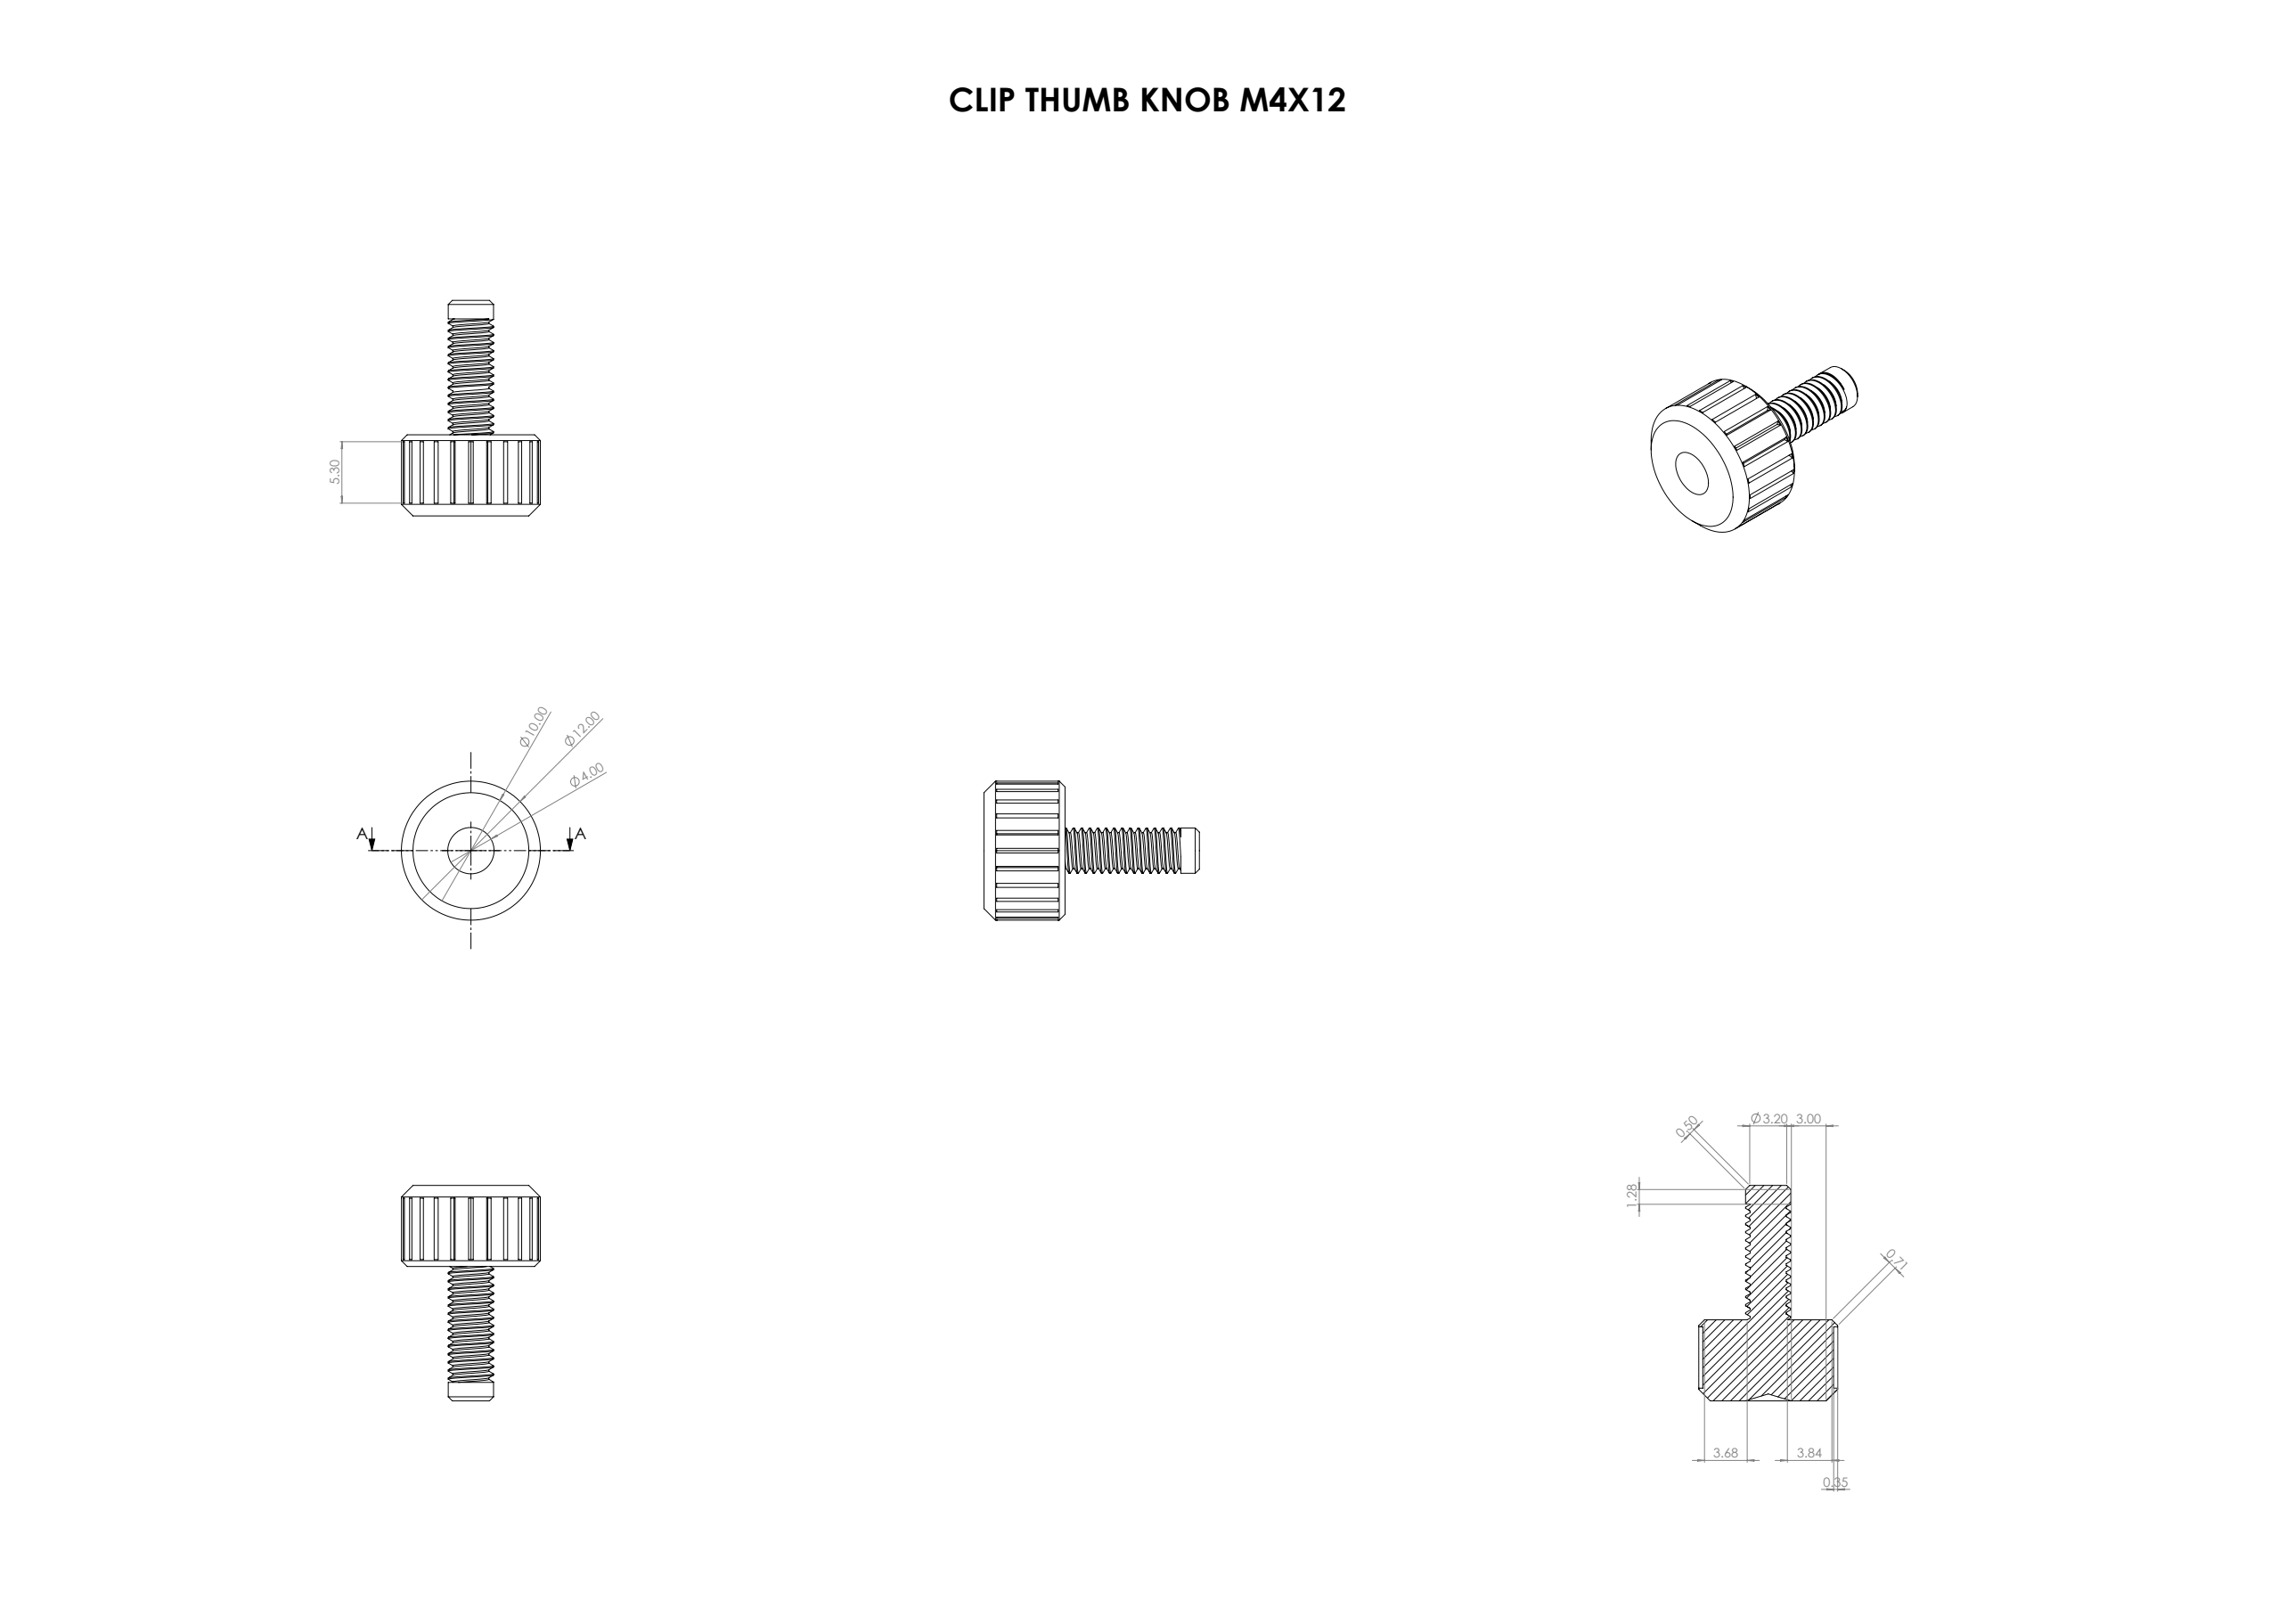
ISO-10303-21;
HEADER;
/* Generated by software containing ST-Developer
 * from STEP Tools, Inc. (www.steptools.com) 
 */

FILE_DESCRIPTION(
/* description */ (''),
/* implementation_level */ '2;1');

FILE_NAME(
/* name */ '11_Clip_Thumb_Knob_M4x12.step',
/* time_stamp */ '2026-10-19T22:59:19-07:00',
/* author */ (''),
/* organization */ (''),
/* preprocessor_version */ 'ST-DEVELOPER v20.2',
/* originating_system */ 'Autodesk Translation Framework v15.15.0.0',
/* authorisation */ '');

FILE_SCHEMA (('AUTOMOTIVE_DESIGN { 1 0 10303 214 3 1 1 }'));
ENDSEC;

DATA;
#10=MECHANICAL_DESIGN_GEOMETRIC_PRESENTATION_REPRESENTATION('',(#923),#53650);
#365=B_SPLINE_SURFACE_WITH_KNOTS('',3,3,((#37203,#37204,#37205,#37206,#37207,
#37208,#37209,#37210,#37211,#37212,#37213,#37214,#37215,#37216,#37217,#37218,
#37219,#37220,#37221,#37222,#37223,#37224,#37225,#37226,#37227,#37228,#37229,
#37230,#37231,#37232,#37233,#37234,#37235,#37236,#37237,#37238,#37239,#37240,
#37241,#37242,#37243,#37244,#37245,#37246,#37247,#37248,#37249,#37250,#37251,
#37252,#37253,#37254,#37255,#37256,#37257,#37258,#37259,#37260,#37261,#37262,
#37263,#37264,#37265,#37266,#37267,#37268,#37269,#37270,#37271,#37272,#37273,
#37274,#37275,#37276,#37277,#37278,#37279,#37280,#37281,#37282,#37283,#37284,
#37285,#37286,#37287,#37288,#37289,#37290,#37291,#37292,#37293,#37294,#37295,
#37296,#37297),(#37298,#37299,#37300,#37301,#37302,#37303,#37304,#37305,
#37306,#37307,#37308,#37309,#37310,#37311,#37312,#37313,#37314,#37315,#37316,
#37317,#37318,#37319,#37320,#37321,#37322,#37323,#37324,#37325,#37326,#37327,
#37328,#37329,#37330,#37331,#37332,#37333,#37334,#37335,#37336,#37337,#37338,
#37339,#37340,#37341,#37342,#37343,#37344,#37345,#37346,#37347,#37348,#37349,
#37350,#37351,#37352,#37353,#37354,#37355,#37356,#37357,#37358,#37359,#37360,
#37361,#37362,#37363,#37364,#37365,#37366,#37367,#37368,#37369,#37370,#37371,
#37372,#37373,#37374,#37375,#37376,#37377,#37378,#37379,#37380,#37381,#37382,
#37383,#37384,#37385,#37386,#37387,#37388,#37389,#37390,#37391,#37392),
(#37393,#37394,#37395,#37396,#37397,#37398,#37399,#37400,#37401,#37402,
#37403,#37404,#37405,#37406,#37407,#37408,#37409,#37410,#37411,#37412,#37413,
#37414,#37415,#37416,#37417,#37418,#37419,#37420,#37421,#37422,#37423,#37424,
#37425,#37426,#37427,#37428,#37429,#37430,#37431,#37432,#37433,#37434,#37435,
#37436,#37437,#37438,#37439,#37440,#37441,#37442,#37443,#37444,#37445,#37446,
#37447,#37448,#37449,#37450,#37451,#37452,#37453,#37454,#37455,#37456,#37457,
#37458,#37459,#37460,#37461,#37462,#37463,#37464,#37465,#37466,#37467,#37468,
#37469,#37470,#37471,#37472,#37473,#37474,#37475,#37476,#37477,#37478,#37479,
#37480,#37481,#37482,#37483,#37484,#37485,#37486,#37487),(#37488,#37489,
#37490,#37491,#37492,#37493,#37494,#37495,#37496,#37497,#37498,#37499,#37500,
#37501,#37502,#37503,#37504,#37505,#37506,#37507,#37508,#37509,#37510,#37511,
#37512,#37513,#37514,#37515,#37516,#37517,#37518,#37519,#37520,#37521,#37522,
#37523,#37524,#37525,#37526,#37527,#37528,#37529,#37530,#37531,#37532,#37533,
#37534,#37535,#37536,#37537,#37538,#37539,#37540,#37541,#37542,#37543,#37544,
#37545,#37546,#37547,#37548,#37549,#37550,#37551,#37552,#37553,#37554,#37555,
#37556,#37557,#37558,#37559,#37560,#37561,#37562,#37563,#37564,#37565,#37566,
#37567,#37568,#37569,#37570,#37571,#37572,#37573,#37574,#37575,#37576,#37577,
#37578,#37579,#37580,#37581,#37582)),.UNSPECIFIED.,.F.,.F.,.F.,(4,4),(4,
1,1,1,1,1,1,1,1,1,1,1,1,1,1,1,1,1,1,1,1,1,1,1,1,1,1,1,1,1,1,1,1,1,1,1,1,
1,1,1,1,1,1,1,1,1,1,1,1,1,1,1,1,1,1,1,1,1,1,1,1,1,1,1,1,1,1,1,1,1,1,1,1,
1,1,1,1,1,1,1,1,1,1,1,1,1,1,1,1,1,1,1,4),(0.,0.0460148164544131),(13.2114714623398,
14.2095685301207,15.2076655979016,16.2057626656825,17.2038597334634,18.2019568012443,
19.2000538690252,20.1981509368061,21.1962480045871,22.194345072368,23.1924421401489,
24.1905392079298,25.1886362757107,26.1867333434916,27.1848304112725,28.1829274790534,
29.1810245468343,30.1791216146152,31.1772186823961,32.1753157501771,33.173412817958,
34.1715098857389,35.1696069535198,36.1677040213007,37.1658010890816,38.1638981568625,
39.1619952246434,40.1600922924243,41.1581893602052,42.1562864279861,43.1543834957671,
44.152480563548,45.1505776313289,46.1486746991098,47.1467717668907,48.1448688346716,
49.1429659024525,50.1410629702334,51.1391600380143,52.1372571057952,53.1353541735761,
54.1334512413571,55.131548309138,56.1296453769189,57.1277424446998,58.1258395124807,
59.1239365802616,60.1220336480425,61.1201307158234,62.1182277836043,63.1163248513852,
64.1144219191661,65.1125189869471,66.110616054728,67.1087131225089,68.1068101902898,
69.1049072580707,70.1030043258516,71.1011013936325,72.0991984614134,73.0972955291943,
74.0953925969752,75.0934896647561,76.0915867325371,77.089683800318,78.0877808680989,
79.0858779358798,80.0839750036607,81.0820720714416,82.0801691392225,83.0782662070034,
84.0763632747843,85.0744603425652,86.0725574103461,87.0706544781271,88.068751545908,
89.0668486136889,90.0649456814698,91.0630427492507,92.0611398170316,93.0592368848125,
94.0573339525934,95.0554310203743,96.0535280881552,97.0516251559362,98.0497222237171,
99.047819291498,100.045916359279,101.04401342706,102.042110494841,103.040207562622,
104.038304630403,105.036401698183),.UNSPECIFIED.);
#366=B_SPLINE_SURFACE_WITH_KNOTS('',3,3,((#37767,#37768,#37769,#37770,#37771,
#37772,#37773,#37774,#37775,#37776,#37777,#37778,#37779,#37780,#37781,#37782,
#37783,#37784,#37785,#37786,#37787,#37788,#37789,#37790,#37791,#37792,#37793,
#37794,#37795,#37796,#37797,#37798,#37799,#37800,#37801,#37802,#37803,#37804,
#37805,#37806,#37807,#37808,#37809,#37810,#37811,#37812,#37813,#37814,#37815,
#37816,#37817,#37818,#37819,#37820,#37821,#37822,#37823,#37824,#37825,#37826,
#37827,#37828,#37829,#37830,#37831,#37832,#37833,#37834,#37835,#37836,#37837,
#37838,#37839,#37840,#37841,#37842,#37843,#37844,#37845,#37846,#37847,#37848,
#37849,#37850,#37851,#37852,#37853,#37854,#37855,#37856,#37857,#37858,#37859,
#37860,#37861),(#37862,#37863,#37864,#37865,#37866,#37867,#37868,#37869,
#37870,#37871,#37872,#37873,#37874,#37875,#37876,#37877,#37878,#37879,#37880,
#37881,#37882,#37883,#37884,#37885,#37886,#37887,#37888,#37889,#37890,#37891,
#37892,#37893,#37894,#37895,#37896,#37897,#37898,#37899,#37900,#37901,#37902,
#37903,#37904,#37905,#37906,#37907,#37908,#37909,#37910,#37911,#37912,#37913,
#37914,#37915,#37916,#37917,#37918,#37919,#37920,#37921,#37922,#37923,#37924,
#37925,#37926,#37927,#37928,#37929,#37930,#37931,#37932,#37933,#37934,#37935,
#37936,#37937,#37938,#37939,#37940,#37941,#37942,#37943,#37944,#37945,#37946,
#37947,#37948,#37949,#37950,#37951,#37952,#37953,#37954,#37955,#37956),
(#37957,#37958,#37959,#37960,#37961,#37962,#37963,#37964,#37965,#37966,
#37967,#37968,#37969,#37970,#37971,#37972,#37973,#37974,#37975,#37976,#37977,
#37978,#37979,#37980,#37981,#37982,#37983,#37984,#37985,#37986,#37987,#37988,
#37989,#37990,#37991,#37992,#37993,#37994,#37995,#37996,#37997,#37998,#37999,
#38000,#38001,#38002,#38003,#38004,#38005,#38006,#38007,#38008,#38009,#38010,
#38011,#38012,#38013,#38014,#38015,#38016,#38017,#38018,#38019,#38020,#38021,
#38022,#38023,#38024,#38025,#38026,#38027,#38028,#38029,#38030,#38031,#38032,
#38033,#38034,#38035,#38036,#38037,#38038,#38039,#38040,#38041,#38042,#38043,
#38044,#38045,#38046,#38047,#38048,#38049,#38050,#38051),(#38052,#38053,
#38054,#38055,#38056,#38057,#38058,#38059,#38060,#38061,#38062,#38063,#38064,
#38065,#38066,#38067,#38068,#38069,#38070,#38071,#38072,#38073,#38074,#38075,
#38076,#38077,#38078,#38079,#38080,#38081,#38082,#38083,#38084,#38085,#38086,
#38087,#38088,#38089,#38090,#38091,#38092,#38093,#38094,#38095,#38096,#38097,
#38098,#38099,#38100,#38101,#38102,#38103,#38104,#38105,#38106,#38107,#38108,
#38109,#38110,#38111,#38112,#38113,#38114,#38115,#38116,#38117,#38118,#38119,
#38120,#38121,#38122,#38123,#38124,#38125,#38126,#38127,#38128,#38129,#38130,
#38131,#38132,#38133,#38134,#38135,#38136,#38137,#38138,#38139,#38140,#38141,
#38142,#38143,#38144,#38145,#38146)),.UNSPECIFIED.,.F.,.F.,.F.,(4,4),(4,
1,1,1,1,1,1,1,1,1,1,1,1,1,1,1,1,1,1,1,1,1,1,1,1,1,1,1,1,1,1,1,1,1,1,1,1,
1,1,1,1,1,1,1,1,1,1,1,1,1,1,1,1,1,1,1,1,1,1,1,1,1,1,1,1,1,1,1,1,1,1,1,1,
1,1,1,1,1,1,1,1,1,1,1,1,1,1,1,1,1,1,1,4),(0.,0.0460148164544131),(16.5163060587106,
17.5144031264916,18.5125001942725,19.5105972620534,20.5086943298343,21.5067913976152,
22.5048884653961,23.502985533177,24.5010826009579,25.4991796687388,26.4972767365197,
27.4953738043006,28.4934708720816,29.4915679398625,30.4896650076434,31.4877620754243,
32.4858591432052,33.4839562109861,34.482053278767,35.4801503465479,36.4782474143288,
37.4763444821097,38.4744415498906,39.4725386176716,40.4706356854525,41.4687327532334,
42.4668298210143,43.4649268887952,44.4630239565761,45.461121024357,46.4592180921379,
47.4573151599188,48.4554122276997,49.4535092954806,50.4516063632615,51.4497034310425,
52.4478004988234,53.4458975666043,54.4439946343852,55.4420917021661,56.440188769947,
57.4382858377279,58.4363829055088,59.4344799732897,60.4325770410706,61.4306741088515,
62.4287711766325,63.4268682444134,64.4249653121943,65.4230623799752,66.4211594477561,
67.419256515537,68.4173535833179,69.4154506510988,70.4135477188797,71.4116447866606,
72.4097418544415,73.4078389222225,74.4059359900034,75.4040330577843,76.4021301255652,
77.4002271933461,78.398324261127,79.3964213289079,80.3945183966888,81.3926154644697,
82.3907125322506,83.3888096000315,84.3869066678125,85.3850037355934,86.3831008033743,
87.3811978711552,88.3792949389361,89.377392006717,90.3754890744979,91.3735861422788,
92.3716832100597,93.3697802778406,94.3678773456216,95.3659744134025,96.3640714811834,
97.3621685489643,98.3602656167452,99.3583626845261,100.356459752307,101.354556820088,
102.352653887869,103.35075095565,104.348848023431,105.346945091212,106.345042158992,
107.343139226773,108.341236294554),.UNSPECIFIED.);
#424=B_SPLINE_CURVE_WITH_KNOTS('',3,(#36162,#36163,#36164,#36165,#36166,
#36167,#36168,#36169,#36170,#36171,#36172,#36173,#36174),.UNSPECIFIED.,
 .F.,.F.,(4,3,3,3,4),(-5.47484251641785,-4.99048533890455,-3.99238827112364,
-2.99429120334273,-2.06514013327811),.UNSPECIFIED.);
#425=B_SPLINE_CURVE_WITH_KNOTS('',3,(#36182,#36183,#36184,#36185,#36186,
#36187,#36188,#36189,#36190,#36191),.UNSPECIFIED.,.F.,.F.,(4,3,3,4),(0.,
0.998097067780899,1.99619413556182,2.49649180560904),.UNSPECIFIED.);
#426=B_SPLINE_CURVE_WITH_KNOTS('',3,(#36196,#36197,#36198,#36199,#36200,
#36201,#36202,#36203,#36204,#36205,#36206,#36207,#36208,#36209,#36210,#36211,
#36212,#36213,#36214,#36215,#36216,#36217),.UNSPECIFIED.,.F.,.F.,(4,3,3,
3,3,3,3,4),(-11.7580278235974,-10.97906774559,-9.9809706778091,-8.98287361002818,
-7.98477654224727,-6.98667947446637,-5.98858240668546,-5.47484251641785),
 .UNSPECIFIED.);
#427=B_SPLINE_CURVE_WITH_KNOTS('',3,(#36218,#36219,#36220,#36221,#36222,
#36223,#36224,#36225,#36226,#36227,#36228,#36229,#36230,#36231,#36232,#36233,
#36234,#36235,#36236,#36237,#36238,#36239),.UNSPECIFIED.,.F.,.F.,(4,3,3,
3,3,3,3,4),(2.49649180560904,2.99429120334273,3.99238827112364,4.99048533890454,
5.98858240668546,6.98667947446636,7.98477654224727,8.77967711278862),
 .UNSPECIFIED.);
#428=B_SPLINE_CURVE_WITH_KNOTS('',3,(#36244,#36245,#36246,#36247,#36248,
#36249,#36250,#36251,#36252,#36253,#36254,#36255,#36256,#36257,#36258,#36259,
#36260,#36261,#36262,#36263,#36264,#36265,#36266,#36267,#36268),
 .UNSPECIFIED.,.F.,.F.,(4,3,3,3,3,3,3,3,4),(-18.041213130777,-17.9657472200564,
-16.9676501522755,-15.9695530844945,-14.9714560167136,-13.9733589489327,
-12.9752618811518,-11.9771648133709,-11.7580278235974),.UNSPECIFIED.);
#429=B_SPLINE_CURVE_WITH_KNOTS('',3,(#36269,#36270,#36271,#36272,#36273,
#36274,#36275,#36276,#36277,#36278,#36279,#36280,#36281,#36282,#36283,#36284,
#36285,#36286,#36287,#36288,#36289,#36290,#36291,#36292,#36293),
 .UNSPECIFIED.,.F.,.F.,(4,3,3,3,3,3,3,3,4),(8.77967711278862,8.98287361002818,
9.98097067780909,10.97906774559,11.9771648133709,12.9752618811518,13.9733589489327,
14.9714560167136,15.0628624199682),.UNSPECIFIED.);
#430=B_SPLINE_CURVE_WITH_KNOTS('',3,(#36298,#36299,#36300,#36301,#36302,
#36303,#36304,#36305,#36306,#36307,#36308,#36309,#36310,#36311,#36312,#36313,
#36314,#36315,#36316,#36317,#36318,#36319),.UNSPECIFIED.,.F.,.F.,(4,3,3,
3,3,3,3,4),(-24.3243984379566,-23.9543296267418,-22.9562325589609,-21.95813549118,
-20.9600384233991,-19.9619413556182,-18.9638442878373,-18.041213130777),
 .UNSPECIFIED.);
#431=B_SPLINE_CURVE_WITH_KNOTS('',3,(#36320,#36321,#36322,#36323,#36324,
#36325,#36326,#36327,#36328,#36329,#36330,#36331,#36332,#36333,#36334,#36335,
#36336,#36337,#36338,#36339,#36340,#36341),.UNSPECIFIED.,.F.,.F.,(4,3,3,
3,3,3,3,4),(15.0628624199682,15.9695530844945,16.9676501522755,17.9657472200564,
18.9638442878373,19.9619413556182,20.9600384233991,21.3460477271478),
 .UNSPECIFIED.);
#432=B_SPLINE_CURVE_WITH_KNOTS('',3,(#36346,#36347,#36348,#36349,#36350,
#36351,#36352,#36353,#36354,#36355,#36356,#36357,#36358,#36359,#36360,#36361,
#36362,#36363,#36364,#36365,#36366,#36367),.UNSPECIFIED.,.F.,.F.,(4,3,3,
3,3,3,3,4),(-30.6075837451362,-29.9429120334273,-28.9448149656464,-27.9467178978655,
-26.9486208300846,-25.9505237623036,-24.9524266945227,-24.3243984379566),
 .UNSPECIFIED.);
#433=B_SPLINE_CURVE_WITH_KNOTS('',3,(#36368,#36369,#36370,#36371,#36372,
#36373,#36374,#36375,#36376,#36377,#36378,#36379,#36380,#36381,#36382,#36383,
#36384,#36385,#36386,#36387,#36388,#36389),.UNSPECIFIED.,.F.,.F.,(4,3,3,
3,3,3,3,4),(21.3460477271478,21.95813549118,22.9562325589609,23.9543296267418,
24.9524266945227,25.9505237623036,26.9486208300845,27.6292330343274),
 .UNSPECIFIED.);
#434=B_SPLINE_CURVE_WITH_KNOTS('',3,(#36394,#36395,#36396,#36397,#36398,
#36399,#36400,#36401,#36402,#36403,#36404,#36405,#36406,#36407,#36408,#36409,
#36410,#36411,#36412,#36413,#36414,#36415),.UNSPECIFIED.,.F.,.F.,(4,3,3,
3,3,3,3,4),(-36.8907690523158,-35.9314944401127,-34.9333973723318,-33.9353003045509,
-32.93720323677,-31.9391061689891,-30.9410091012082,-30.6075837451362),
 .UNSPECIFIED.);
#435=B_SPLINE_CURVE_WITH_KNOTS('',3,(#36416,#36417,#36418,#36419,#36420,
#36421,#36422,#36423,#36424,#36425,#36426,#36427,#36428,#36429,#36430,#36431,
#36432,#36433,#36434,#36435,#36436,#36437),.UNSPECIFIED.,.F.,.F.,(4,3,3,
3,3,3,3,4),(27.6292330343274,27.9467178978654,28.9448149656464,29.9429120334273,
30.9410091012082,31.9391061689891,32.93720323677,33.912418341507),
 .UNSPECIFIED.);
#436=B_SPLINE_CURVE_WITH_KNOTS('',3,(#36442,#36443,#36444,#36445,#36446,
#36447,#36448,#36449,#36450,#36451,#36452,#36453,#36454,#36455,#36456,#36457,
#36458,#36459,#36460,#36461,#36462,#36463,#36464,#36465,#36466),
 .UNSPECIFIED.,.F.,.F.,(4,3,3,3,3,3,3,3,4),(-43.1739543594954,-42.9181739145791,
-41.9200768467982,-40.9219797790173,-39.9238827112364,-38.9257856434555,
-37.9276885756746,-36.9295915078936,-36.8907690523158),.UNSPECIFIED.);
#437=B_SPLINE_CURVE_WITH_KNOTS('',3,(#36467,#36468,#36469,#36470,#36471,
#36472,#36473,#36474,#36475,#36476,#36477,#36478,#36479,#36480,#36481,#36482,
#36483,#36484,#36485,#36486,#36487,#36488,#36489,#36490,#36491),
 .UNSPECIFIED.,.F.,.F.,(4,3,3,3,3,3,3,3,4),(33.912418341507,33.9353003045509,
34.9333973723318,35.9314944401127,36.9295915078936,37.9276885756745,38.9257856434555,
39.9238827112364,40.1956036486866),.UNSPECIFIED.);
#438=B_SPLINE_CURVE_WITH_KNOTS('',3,(#36496,#36497,#36498,#36499,#36500,
#36501,#36502,#36503,#36504,#36505,#36506,#36507,#36508,#36509,#36510,#36511,
#36512,#36513,#36514,#36515,#36516,#36517),.UNSPECIFIED.,.F.,.F.,(4,3,3,
3,3,3,3,4),(-49.457139666675,-48.9067563212645,-47.9086592534836,-46.9105621857027,
-45.9124651179218,-44.9143680501409,-43.91627098236,-43.1739543594954),
 .UNSPECIFIED.);
#439=B_SPLINE_CURVE_WITH_KNOTS('',3,(#36518,#36519,#36520,#36521,#36522,
#36523,#36524,#36525,#36526,#36527,#36528,#36529,#36530,#36531,#36532,#36533,
#36534,#36535,#36536,#36537,#36538,#36539),.UNSPECIFIED.,.F.,.F.,(4,3,3,
3,3,3,3,4),(40.1956036486866,40.9219797790173,41.9200768467982,42.9181739145791,
43.91627098236,44.9143680501409,45.9124651179218,46.4787889558661),
 .UNSPECIFIED.);
#440=B_SPLINE_CURVE_WITH_KNOTS('',3,(#36544,#36545,#36546,#36547,#36548,
#36549,#36550,#36551,#36552,#36553,#36554,#36555,#36556,#36557,#36558,#36559,
#36560,#36561,#36562,#36563,#36564,#36565),.UNSPECIFIED.,.F.,.F.,(4,3,3,
3,3,3,3,4),(-55.7403249738546,-54.89533872795,-53.8972416601691,-52.8991445923882,
-51.9010475246073,-50.9029504568264,-49.9048533890454,-49.457139666675),
 .UNSPECIFIED.);
#441=B_SPLINE_CURVE_WITH_KNOTS('',3,(#36566,#36567,#36568,#36569,#36570,
#36571,#36572,#36573,#36574,#36575,#36576,#36577,#36578,#36579,#36580,#36581,
#36582,#36583,#36584,#36585,#36586,#36587),.UNSPECIFIED.,.F.,.F.,(4,3,3,
3,3,3,3,4),(46.4787889558661,46.9105621857027,47.9086592534836,48.9067563212645,
49.9048533890454,50.9029504568264,51.9010475246073,52.7619742630458),
 .UNSPECIFIED.);
#442=B_SPLINE_CURVE_WITH_KNOTS('',3,(#36592,#36593,#36594,#36595,#36596,
#36597,#36598,#36599,#36600,#36601,#36602,#36603,#36604,#36605,#36606,#36607,
#36608,#36609,#36610,#36611,#36612,#36613,#36614,#36615,#36616),
 .UNSPECIFIED.,.F.,.F.,(4,3,3,3,3,3,3,3,4),(-62.0235102810341,-61.8820182024164,
-60.8839211346355,-59.8858240668546,-58.8877269990736,-57.8896299312927,
-56.8915328635118,-55.8934357957309,-55.7403249738546),.UNSPECIFIED.);
#443=B_SPLINE_CURVE_WITH_KNOTS('',3,(#36617,#36618,#36619,#36620,#36621,
#36622,#36623,#36624,#36625,#36626,#36627,#36628,#36629,#36630,#36631,#36632,
#36633,#36634,#36635,#36636,#36637,#36638,#36639,#36640,#36641),
 .UNSPECIFIED.,.F.,.F.,(4,3,3,3,3,3,3,3,4),(52.7619742630458,52.8991445923882,
53.8972416601691,54.89533872795,55.8934357957309,56.8915328635118,57.8896299312927,
58.8877269990736,59.0451595702253),.UNSPECIFIED.);
#444=B_SPLINE_CURVE_WITH_KNOTS('',3,(#36646,#36647,#36648,#36649,#36650,
#36651,#36652,#36653,#36654,#36655,#36656,#36657,#36658,#36659,#36660,#36661,
#36662,#36663,#36664,#36665,#36666,#36667),.UNSPECIFIED.,.F.,.F.,(4,3,3,
3,3,3,3,4),(-68.3066955882137,-67.8706006091018,-66.8725035413209,-65.87440647354,
-64.8763094057591,-63.8782123379782,-62.8801152701973,-62.0235102810341),
 .UNSPECIFIED.);
#445=B_SPLINE_CURVE_WITH_KNOTS('',3,(#36668,#36669,#36670,#36671,#36672,
#36673,#36674,#36675,#36676,#36677,#36678,#36679,#36680,#36681,#36682,#36683,
#36684,#36685,#36686,#36687,#36688,#36689),.UNSPECIFIED.,.F.,.F.,(4,3,3,
3,3,3,3,4),(59.0451595702253,59.8858240668545,60.8839211346355,61.8820182024164,
62.8801152701973,63.8782123379782,64.8763094057591,65.3283448774049),
 .UNSPECIFIED.);
#446=B_SPLINE_CURVE_WITH_KNOTS('',3,(#36694,#36695,#36696,#36697,#36698,
#36699,#36700,#36701,#36702,#36703,#36704,#36705,#36706,#36707,#36708,#36709,
#36710,#36711,#36712,#36713,#36714,#36715),.UNSPECIFIED.,.F.,.F.,(4,3,3,
3,3,3,3,4),(-74.5898808953933,-73.8591830157873,-72.8610859480063,-71.8629888802254,
-70.8648918124445,-69.8667947446636,-68.8686976768827,-68.3066955882137),
 .UNSPECIFIED.);
#447=B_SPLINE_CURVE_WITH_KNOTS('',3,(#36716,#36717,#36718,#36719,#36720,
#36721,#36722,#36723,#36724,#36725,#36726,#36727,#36728,#36729,#36730,#36731,
#36732,#36733,#36734,#36735,#36736,#36737),.UNSPECIFIED.,.F.,.F.,(4,3,3,
3,3,3,3,4),(65.3283448774049,65.87440647354,66.8725035413209,67.8706006091018,
68.8686976768827,69.8667947446636,70.8648918124445,71.6115301845845),
 .UNSPECIFIED.);
#448=B_SPLINE_CURVE_WITH_KNOTS('',3,(#36742,#36743,#36744,#36745,#36746,
#36747,#36748,#36749,#36750,#36751,#36752,#36753,#36754,#36755,#36756,#36757,
#36758,#36759,#36760,#36761,#36762,#36763,#36764,#36765,#36766),
 .UNSPECIFIED.,.F.,.F.,(4,3,3,3,3,3,3,3,4),(-80.8730662025729,-80.8458624902537,
-79.8477654224727,-78.8496683546918,-77.8515712869109,-76.85347421913,-75.8553771513491,
-74.8572800835682,-74.5898808953933),.UNSPECIFIED.);
#449=B_SPLINE_CURVE_WITH_KNOTS('',3,(#36767,#36768,#36769,#36770,#36771,
#36772,#36773,#36774,#36775,#36776,#36777,#36778,#36779,#36780,#36781,#36782,
#36783,#36784,#36785,#36786,#36787,#36788,#36789,#36790,#36791),
 .UNSPECIFIED.,.F.,.F.,(4,3,3,3,3,3,3,3,4),(71.6115301845845,71.8629888802254,
72.8610859480063,73.8591830157873,74.8572800835682,75.8553771513491,76.85347421913,
77.8515712869109,77.8947154917641),.UNSPECIFIED.);
#450=B_SPLINE_CURVE_WITH_KNOTS('',3,(#36796,#36797,#36798,#36799,#36800,
#36801,#36802,#36803,#36804,#36805,#36806,#36807,#36808,#36809,#36810,#36811,
#36812,#36813,#36814,#36815,#36816,#36817),.UNSPECIFIED.,.F.,.F.,(4,3,3,
3,3,3,3,4),(-87.1562515097525,-86.8344448969391,-85.8363478291582,-84.8382507613773,
-83.8401536935964,-82.8420566258155,-81.8439595580345,-80.8730662025729),
 .UNSPECIFIED.);
#451=B_SPLINE_CURVE_WITH_KNOTS('',3,(#36818,#36819,#36820,#36821,#36822,
#36823,#36824,#36825,#36826,#36827,#36828,#36829,#36830,#36831,#36832,#36833,
#36834,#36835,#36836,#36837,#36838,#36839),.UNSPECIFIED.,.F.,.F.,(4,3,3,
3,3,3,3,4),(77.8947154917641,78.8496683546918,79.8477654224727,80.8458624902536,
81.8439595580346,82.8420566258154,83.8401536935964,84.1779007989437),
 .UNSPECIFIED.);
#452=B_SPLINE_CURVE_WITH_KNOTS('',3,(#36845,#36846,#36847,#36848,#36849,
#36850),.UNSPECIFIED.,.F.,.F.,(4,1,1,4),(103.672557568463,104.348848023431,
105.346945091212,106.276096161276),.UNSPECIFIED.);
#453=B_SPLINE_CURVE_WITH_KNOTS('',3,(#36853,#36854,#36855,#36856,#36857),
 .UNSPECIFIED.,.F.,.F.,(4,1,4),(103.672557568463,104.038304630403,105.036401698183),
 .UNSPECIFIED.);
#454=B_SPLINE_CURVE_WITH_KNOTS('',3,(#36862,#36863,#36864,#36865,#36866,
#36867,#36868,#36869,#36870,#36871),.UNSPECIFIED.,.F.,.F.,(4,1,1,1,1,1,
1,4),(97.3893722612836,98.3602656167452,99.3583626845261,100.356459752307,
101.354556820088,102.352653887869,103.35075095565,103.672557568463),
 .UNSPECIFIED.);
#455=B_SPLINE_CURVE_WITH_KNOTS('',3,(#36872,#36873,#36874,#36875,#36876,
#36877,#36878,#36879,#36880,#36881),.UNSPECIFIED.,.F.,.F.,(4,1,1,1,1,1,
1,4),(97.3893722612836,98.0497222237171,99.047819291498,100.045916359279,
101.04401342706,102.042110494841,103.040207562622,103.672557568463),
 .UNSPECIFIED.);
#456=B_SPLINE_CURVE_WITH_KNOTS('',3,(#36886,#36887,#36888,#36889,#36890,
#36891,#36892,#36893,#36894,#36895,#36896),.UNSPECIFIED.,.F.,.F.,(4,1,1,
1,1,1,1,1,4),(91.106186954104,91.3735861422788,92.3716832100597,93.3697802778406,
94.3678773456216,95.3659744134025,96.3640714811834,97.3621685489643,97.3893722612836),
 .UNSPECIFIED.);
#457=B_SPLINE_CURVE_WITH_KNOTS('',3,(#36897,#36898,#36899,#36900,#36901,
#36902,#36903,#36904,#36905,#36906),.UNSPECIFIED.,.F.,.F.,(4,1,1,1,1,1,
1,4),(91.106186954104,92.0611398170316,93.0592368848125,94.0573339525934,
95.0554310203743,96.0535280881552,97.0516251559362,97.3893722612836),
 .UNSPECIFIED.);
#458=B_SPLINE_CURVE_WITH_KNOTS('',3,(#36911,#36912,#36913,#36914,#36915,
#36916,#36917,#36918,#36919,#36920),.UNSPECIFIED.,.F.,.F.,(4,1,1,1,1,1,
1,4),(84.8230016469244,85.3850037355934,86.3831008033743,87.3811978711552,
88.3792949389361,89.377392006717,90.3754890744979,91.106186954104),
 .UNSPECIFIED.);
#459=B_SPLINE_CURVE_WITH_KNOTS('',3,(#36921,#36922,#36923,#36924,#36925,
#36926,#36927,#36928,#36929,#36930,#36931),.UNSPECIFIED.,.F.,.F.,(4,1,1,
1,1,1,1,1,4),(84.8230016469244,85.0744603425652,86.0725574103461,87.0706544781271,
88.068751545908,89.0668486136889,90.0649456814698,91.0630427492507,91.106186954104),
 .UNSPECIFIED.);
#460=B_SPLINE_CURVE_WITH_KNOTS('',3,(#36936,#36937,#36938,#36939,#36940,
#36941,#36942,#36943,#36944,#36945),.UNSPECIFIED.,.F.,.F.,(4,1,1,1,1,1,
1,4),(78.5398163397448,79.3964213289079,80.3945183966888,81.3926154644697,
82.3907125322506,83.3888096000315,84.3869066678125,84.8230016469244),
 .UNSPECIFIED.);
#461=B_SPLINE_CURVE_WITH_KNOTS('',3,(#36946,#36947,#36948,#36949,#36950,
#36951,#36952,#36953,#36954,#36955),.UNSPECIFIED.,.F.,.F.,(4,1,1,1,1,1,
1,4),(78.5398163397448,79.0858779358798,80.0839750036607,81.0820720714416,
82.0801691392225,83.0782662070034,84.0763632747843,84.8230016469244),
 .UNSPECIFIED.);
#462=B_SPLINE_CURVE_WITH_KNOTS('',3,(#36960,#36961,#36962,#36963,#36964,
#36965,#36966,#36967,#36968,#36969,#36970),.UNSPECIFIED.,.F.,.F.,(4,1,1,
1,1,1,1,1,4),(72.2566310325652,72.4097418544415,73.4078389222225,74.4059359900034,
75.4040330577843,76.4021301255652,77.4002271933461,78.398324261127,78.5398163397448),
 .UNSPECIFIED.);
#463=B_SPLINE_CURVE_WITH_KNOTS('',3,(#36971,#36972,#36973,#36974,#36975,
#36976,#36977,#36978,#36979,#36980),.UNSPECIFIED.,.F.,.F.,(4,1,1,1,1,1,
1,4),(72.2566310325652,73.0972955291943,74.0953925969752,75.0934896647561,
76.0915867325371,77.089683800318,78.0877808680989,78.5398163397448),
 .UNSPECIFIED.);
#464=B_SPLINE_CURVE_WITH_KNOTS('',3,(#36985,#36986,#36987,#36988,#36989,
#36990,#36991,#36992,#36993,#36994),.UNSPECIFIED.,.F.,.F.,(4,1,1,1,1,1,
1,4),(65.9734457253856,66.4211594477561,67.419256515537,68.4173535833179,
69.4154506510988,70.4135477188797,71.4116447866606,72.2566310325652),
 .UNSPECIFIED.);
#465=B_SPLINE_CURVE_WITH_KNOTS('',3,(#36995,#36996,#36997,#36998,#36999,
#37000,#37001,#37002,#37003,#37004,#37005),.UNSPECIFIED.,.F.,.F.,(4,1,1,
1,1,1,1,1,4),(65.9734457253856,66.110616054728,67.1087131225089,68.1068101902898,
69.1049072580707,70.1030043258516,71.1011013936325,72.0991984614134,72.2566310325652),
 .UNSPECIFIED.);
#466=B_SPLINE_CURVE_WITH_KNOTS('',3,(#37010,#37011,#37012,#37013,#37014,
#37015,#37016,#37017,#37018,#37019),.UNSPECIFIED.,.F.,.F.,(4,1,1,1,1,1,
1,4),(59.690260418206,60.4325770410706,61.4306741088515,62.4287711766325,
63.4268682444134,64.4249653121943,65.4230623799752,65.9734457253856),
 .UNSPECIFIED.);
#467=B_SPLINE_CURVE_WITH_KNOTS('',3,(#37020,#37021,#37022,#37023,#37024,
#37025,#37026,#37027,#37028,#37029),.UNSPECIFIED.,.F.,.F.,(4,1,1,1,1,1,
1,4),(59.690260418206,60.1220336480425,61.1201307158234,62.1182277836043,
63.1163248513852,64.1144219191661,65.1125189869471,65.9734457253856),
 .UNSPECIFIED.);
#468=B_SPLINE_CURVE_WITH_KNOTS('',3,(#37034,#37035,#37036,#37037,#37038,
#37039,#37040,#37041,#37042,#37043,#37044),.UNSPECIFIED.,.F.,.F.,(4,1,1,
1,1,1,1,1,4),(53.4070751110265,53.4458975666043,54.4439946343852,55.4420917021661,
56.440188769947,57.4382858377279,58.4363829055088,59.4344799732897,59.690260418206),
 .UNSPECIFIED.);
#469=B_SPLINE_CURVE_WITH_KNOTS('',3,(#37045,#37046,#37047,#37048,#37049,
#37050,#37051,#37052,#37053,#37054),.UNSPECIFIED.,.F.,.F.,(4,1,1,1,1,1,
1,4),(53.4070751110264,54.1334512413571,55.131548309138,56.1296453769189,
57.1277424446998,58.1258395124807,59.1239365802616,59.690260418206),
 .UNSPECIFIED.);
#470=B_SPLINE_CURVE_WITH_KNOTS('',3,(#37059,#37060,#37061,#37062,#37063,
#37064,#37065,#37066,#37067,#37068),.UNSPECIFIED.,.F.,.F.,(4,1,1,1,1,1,
1,4),(47.1238898038469,47.4573151599188,48.4554122276997,49.4535092954806,
50.4516063632615,51.4497034310425,52.4478004988234,53.4070751110265),
 .UNSPECIFIED.);
#471=B_SPLINE_CURVE_WITH_KNOTS('',3,(#37069,#37070,#37071,#37072,#37073,
#37074,#37075,#37076,#37077,#37078,#37079),.UNSPECIFIED.,.F.,.F.,(4,1,1,
1,1,1,1,1,4),(47.1238898038468,47.1467717668907,48.1448688346716,49.1429659024525,
50.1410629702334,51.1391600380143,52.1372571057952,53.1353541735761,53.4070751110264),
 .UNSPECIFIED.);
#472=B_SPLINE_CURVE_WITH_KNOTS('',3,(#37084,#37085,#37086,#37087,#37088,
#37089,#37090,#37091,#37092,#37093),.UNSPECIFIED.,.F.,.F.,(4,1,1,1,1,1,
1,4),(40.8407044966673,41.4687327532334,42.4668298210143,43.4649268887952,
44.4630239565761,45.461121024357,46.4592180921379,47.1238898038469),
 .UNSPECIFIED.);
#473=B_SPLINE_CURVE_WITH_KNOTS('',3,(#37094,#37095,#37096,#37097,#37098,
#37099,#37100,#37101,#37102,#37103),.UNSPECIFIED.,.F.,.F.,(4,1,1,1,1,1,
1,4),(40.8407044966673,41.1581893602052,42.1562864279861,43.1543834957671,
44.152480563548,45.1505776313289,46.1486746991098,47.1238898038468),
 .UNSPECIFIED.);
#474=B_SPLINE_CURVE_WITH_KNOTS('',3,(#37108,#37109,#37110,#37111,#37112,
#37113,#37114,#37115,#37116,#37117),.UNSPECIFIED.,.F.,.F.,(4,1,1,1,1,1,
1,4),(34.5575191894877,35.4801503465479,36.4782474143288,37.4763444821097,
38.4744415498906,39.4725386176716,40.4706356854525,40.8407044966673),
 .UNSPECIFIED.);
#475=B_SPLINE_CURVE_WITH_KNOTS('',3,(#37118,#37119,#37120,#37121,#37122,
#37123,#37124,#37125,#37126,#37127),.UNSPECIFIED.,.F.,.F.,(4,1,1,1,1,1,
1,4),(34.5575191894876,35.1696069535198,36.1677040213007,37.1658010890816,
38.1638981568625,39.1619952246434,40.1600922924243,40.8407044966673),
 .UNSPECIFIED.);
#476=B_SPLINE_CURVE_WITH_KNOTS('',3,(#37132,#37133,#37134,#37135,#37136,
#37137,#37138,#37139,#37140,#37141,#37142),.UNSPECIFIED.,.F.,.F.,(4,1,1,
1,1,1,1,1,4),(28.2743338823081,28.4934708720816,29.4915679398625,30.4896650076434,
31.4877620754243,32.4858591432052,33.4839562109861,34.482053278767,34.5575191894877),
 .UNSPECIFIED.);
#477=B_SPLINE_CURVE_WITH_KNOTS('',3,(#37143,#37144,#37145,#37146,#37147,
#37148,#37149,#37150,#37151,#37152),.UNSPECIFIED.,.F.,.F.,(4,1,1,1,1,1,
1,4),(28.2743338823081,29.1810245468343,30.1791216146152,31.1772186823961,
32.1753157501771,33.173412817958,34.1715098857389,34.5575191894876),
 .UNSPECIFIED.);
#478=B_SPLINE_CURVE_WITH_KNOTS('',3,(#37157,#37158,#37159,#37160,#37161,
#37162,#37163,#37164,#37165,#37166),.UNSPECIFIED.,.F.,.F.,(4,1,1,1,1,1,
1,4),(21.9911485751285,22.5048884653961,23.502985533177,24.5010826009579,
25.4991796687388,26.4972767365197,27.4953738043006,28.2743338823081),
 .UNSPECIFIED.);
#479=B_SPLINE_CURVE_WITH_KNOTS('',3,(#37167,#37168,#37169,#37170,#37171,
#37172,#37173,#37174,#37175,#37176,#37177),.UNSPECIFIED.,.F.,.F.,(4,1,1,
1,1,1,1,1,4),(21.9911485751285,22.194345072368,23.1924421401489,24.1905392079298,
25.1886362757107,26.1867333434916,27.1848304112725,28.1829274790534,28.2743338823081),
 .UNSPECIFIED.);
#480=B_SPLINE_CURVE_WITH_KNOTS('',3,(#37184,#37185,#37186,#37187,#37188,
#37189,#37190,#37191,#37192),.UNSPECIFIED.,.F.,.F.,(4,1,1,1,1,1,4),(16.5163060587106,
17.5144031264916,18.5125001942725,19.5105972620534,20.5086943298343,21.5067913976152,
21.9911485751285),.UNSPECIFIED.);
#481=B_SPLINE_CURVE_WITH_KNOTS('',3,(#37193,#37194,#37195,#37196,#37197,
#37198,#37199,#37200,#37201,#37202),.UNSPECIFIED.,.F.,.F.,(4,1,1,1,1,1,
1,4),(15.7079632679489,16.2057626656825,17.2038597334634,18.2019568012443,
19.2000538690252,20.1981509368061,21.1962480045871,21.9911485751285),
 .UNSPECIFIED.);
#482=B_SPLINE_CURVE_WITH_KNOTS('',3,(#37584,#37585,#37586,#37587,#37588,
#37589,#37590,#37591,#37592,#37593,#37594,#37595,#37596,#37597,#37598,#37599,
#37600,#37601,#37602,#37603,#37604,#37605,#37606,#37607,#37608,#37609,#37610,
#37611,#37612,#37613,#37614,#37615,#37616,#37617,#37618,#37619,#37620,#37621,
#37622,#37623,#37624,#37625,#37626,#37627,#37628,#37629,#37630,#37631,#37632,
#37633,#37634,#37635),.UNSPECIFIED.,.F.,.F.,(4,3,3,3,3,3,3,3,3,3,3,3,3,
3,3,3,3,4),(-0.364629307890681,-0.351181914845152,-0.324753851954228,-0.31145962862552,
-0.274713453807112,-0.262559121200167,-0.225887319857606,-0.201681225023098,
-0.18621980244873,-0.166307755252122,-0.130572805038765,-0.119339783412349,
-0.0895048375592621,-0.072935651299665,-0.0625561387419937,-0.0518706549961582,
-0.019619443813511,0.),.UNSPECIFIED.);
#483=B_SPLINE_CURVE_WITH_KNOTS('',3,(#37636,#37637,#37638,#37639,#37640,
#37641,#37642,#37643,#37644,#37645,#37646,#37647,#37648,#37649,#37650,#37651,
#37652,#37653,#37654),.UNSPECIFIED.,.F.,.F.,(4,3,3,3,3,3,4),(84.1779007989437,
84.8382507613773,85.8363478291582,86.8344448969391,87.83254196472,88.8306390325009,
89.7597901025655),.UNSPECIFIED.);
#484=B_SPLINE_CURVE_WITH_KNOTS('',3,(#37656,#37657,#37658,#37659,#37660,
#37661,#37662,#37663,#37664,#37665,#37666,#37667,#37668,#37669,#37670,#37671,
#37672,#37673,#37674,#37675,#37676,#37677,#37678,#37679,#37680,#37681,#37682,
#37683,#37684,#37685,#37686,#37687,#37688,#37689,#37690,#37691,#37692,#37693,
#37694,#37695,#37696,#37697,#37698,#37699,#37700,#37701,#37702,#37703,#37704,
#37705,#37706,#37707),.UNSPECIFIED.,.F.,.F.,(4,3,3,3,3,3,3,3,3,3,3,3,3,
3,3,3,3,4),(-0.36639757900585,-0.355489874273349,-0.328849435073975,-0.31597973424817,
-0.292469703717351,-0.280219243073488,-0.245242540668626,-0.218587119974093,
-0.20792985214368,-0.187225496763673,-0.163822309668214,-0.149605700274317,
-0.13878185835336,-0.10408639376502,-0.0828199205047292,-0.0667724235854585,
-0.0282787680692534,0.),.UNSPECIFIED.);
#485=B_SPLINE_CURVE_WITH_KNOTS('',3,(#37708,#37709,#37710,#37711),
 .UNSPECIFIED.,.F.,.F.,(4,4),(15.2766115956179,15.7079632679489),
 .UNSPECIFIED.);
#486=B_SPLINE_CURVE_WITH_KNOTS('',3,(#37713,#37714,#37715,#37716,#37717,
#37718,#37719,#37720,#37721,#37722,#37723,#37724,#37725,#37726,#37727,#37728,
#37729,#37730,#37731,#37732,#37733,#37734,#37735,#37736,#37737,#37738,#37739,
#37740,#37741,#37742,#37743,#37744,#37745,#37746,#37747,#37748,#37749,#37750,
#37751,#37752,#37753,#37754,#37755,#37756,#37757,#37758,#37759,#37760,#37761,
#37762,#37763,#37764),.UNSPECIFIED.,.F.,.F.,(4,3,3,3,3,3,3,3,3,3,3,3,3,
3,3,3,3,4),(-0.36462930789066,-0.351181914845128,-0.324753847158882,-0.311459613184419,
-0.27471342084418,-0.262559086408708,-0.225887280111663,-0.20168112730567,
-0.18621981366523,-0.166307755252114,-0.130572803308094,-0.119339784451787,
-0.0895048383388406,-0.072935654322955,-0.0625561487919195,-0.0518706577021471,
-0.0196194685578637,0.),.UNSPECIFIED.);
#487=B_SPLINE_CURVE_WITH_KNOTS('',3,(#38148,#38149,#38150,#38151,#38152,
#38153,#38154,#38155,#38156,#38157,#38158,#38159,#38160,#38161,#38162,#38163,
#38164,#38165,#38166,#38167,#38168,#38169,#38170,#38171,#38172,#38173,#38174,
#38175,#38176,#38177,#38178,#38179,#38180,#38181,#38182,#38183,#38184,#38185,
#38186,#38187,#38188,#38189,#38190,#38191,#38192,#38193,#38194,#38195,#38196,
#38197,#38198,#38199),.UNSPECIFIED.,.F.,.F.,(4,3,3,3,3,3,3,3,3,3,3,3,3,
3,3,3,3,4),(-0.366397579005837,-0.355489874273339,-0.328849434310144,-0.315979731231902,
-0.292469839731824,-0.280219291818356,-0.245242586893988,-0.218587212262585,
-0.207929893305042,-0.187225496763668,-0.16382230966821,-0.149605709635192,
-0.138781865725635,-0.104086399294226,-0.0828199340175651,-0.0667724231415902,
-0.0282787740817212,0.),.UNSPECIFIED.);
#488=B_SPLINE_CURVE_WITH_KNOTS('',3,(#38200,#38201,#38202,#38203,#38204,
#38205,#38206,#38207,#38208,#38209,#38210,#38211,#38212,#38213,#38214,#38215),
 .UNSPECIFIED.,.F.,.F.,(4,3,3,3,3,4),(-91.8249302358436,-90.8268331680627,
-89.8287361002818,-88.8306390325009,-87.83254196472,-87.1562515097525),
 .UNSPECIFIED.);
#891=SHAPE_REPRESENTATION_RELATIONSHIP('SRR','None',#53736,#907);
#907=ADVANCED_BREP_SHAPE_REPRESENTATION('',(#939),#53646);
#923=STYLED_ITEM('',(#53944),#939);
#939=MANIFOLD_SOLID_BREP('Thumb Knob',#23315);
#1053=CYLINDRICAL_SURFACE('',#24596,0.1954);
#1054=CYLINDRICAL_SURFACE('',#24600,0.1954);
#1055=CYLINDRICAL_SURFACE('',#24601,0.1954);
#1056=CYLINDRICAL_SURFACE('',#24602,0.1954);
#1057=CYLINDRICAL_SURFACE('',#24603,0.1954);
#1058=CYLINDRICAL_SURFACE('',#24604,0.1954);
#1059=CYLINDRICAL_SURFACE('',#24605,0.1954);
#1060=CYLINDRICAL_SURFACE('',#24606,0.1954);
#1061=CYLINDRICAL_SURFACE('',#24607,0.1954);
#1062=CYLINDRICAL_SURFACE('',#24608,0.1954);
#1063=CYLINDRICAL_SURFACE('',#24609,0.1954);
#1064=CYLINDRICAL_SURFACE('',#24610,0.1954);
#1065=CYLINDRICAL_SURFACE('',#24611,0.1954);
#1066=CYLINDRICAL_SURFACE('',#24612,0.1954);
#1067=CYLINDRICAL_SURFACE('',#24613,0.15555);
#1068=CYLINDRICAL_SURFACE('',#24615,0.15555);
#1069=CYLINDRICAL_SURFACE('',#24616,0.15555);
#1070=CYLINDRICAL_SURFACE('',#24617,0.15555);
#1071=CYLINDRICAL_SURFACE('',#24618,0.15555);
#1072=CYLINDRICAL_SURFACE('',#24619,0.15555);
#1073=CYLINDRICAL_SURFACE('',#24620,0.15555);
#1074=CYLINDRICAL_SURFACE('',#24621,0.15555);
#1075=CYLINDRICAL_SURFACE('',#24622,0.15555);
#1076=CYLINDRICAL_SURFACE('',#24623,0.15555);
#1077=CYLINDRICAL_SURFACE('',#24624,0.15555);
#1078=CYLINDRICAL_SURFACE('',#24625,0.15555);
#1079=CYLINDRICAL_SURFACE('',#24626,0.15555);
#1080=CYLINDRICAL_SURFACE('',#24627,0.15555);
#1081=CYLINDRICAL_SURFACE('',#24628,0.15555);
#1082=CYLINDRICAL_SURFACE('',#24632,0.15555);
#1083=CYLINDRICAL_SURFACE('',#24633,0.1954);
#1084=CYLINDRICAL_SURFACE('',#24790,0.6);
#1414=FACE_BOUND('',#4455,.T.);
#1415=FACE_BOUND('',#4458,.T.);
#1416=FACE_BOUND('',#4459,.T.);
#1417=FACE_BOUND('',#4460,.T.);
#1418=FACE_BOUND('',#4461,.T.);
#1419=FACE_BOUND('',#4462,.T.);
#1420=FACE_BOUND('',#4463,.T.);
#1421=FACE_BOUND('',#4464,.T.);
#1422=FACE_BOUND('',#4465,.T.);
#1423=FACE_BOUND('',#4466,.T.);
#1424=FACE_BOUND('',#4467,.T.);
#1425=FACE_BOUND('',#4468,.T.);
#1426=FACE_BOUND('',#4469,.T.);
#1427=FACE_BOUND('',#4470,.T.);
#1428=FACE_BOUND('',#4471,.T.);
#1429=FACE_BOUND('',#4472,.T.);
#1430=FACE_BOUND('',#4473,.T.);
#1431=FACE_BOUND('',#4474,.T.);
#1432=FACE_BOUND('',#4475,.T.);
#1433=FACE_BOUND('',#4476,.T.);
#1434=FACE_BOUND('',#4477,.T.);
#1435=FACE_BOUND('',#4478,.T.);
#1436=FACE_BOUND('',#4479,.T.);
#1437=FACE_BOUND('',#4480,.T.);
#1438=FACE_BOUND('',#4483,.T.);
#1776=PLANE('',#24630);
#1777=PLANE('',#24637);
#1778=PLANE('',#24638);
#1779=PLANE('',#24640);
#1780=PLANE('',#24641);
#1781=PLANE('',#24643);
#1782=PLANE('',#24644);
#1783=PLANE('',#24646);
#1784=PLANE('',#24647);
#1785=PLANE('',#24649);
#1786=PLANE('',#24650);
#1787=PLANE('',#24652);
#1788=PLANE('',#24653);
#1789=PLANE('',#24655);
#1790=PLANE('',#24656);
#1791=PLANE('',#24658);
#1792=PLANE('',#24659);
#1793=PLANE('',#24661);
#1794=PLANE('',#24662);
#1795=PLANE('',#24664);
#1796=PLANE('',#24665);
#1797=PLANE('',#24667);
#1798=PLANE('',#24668);
#1799=PLANE('',#24670);
#1800=PLANE('',#24671);
#1801=PLANE('',#24673);
#1802=PLANE('',#24674);
#1803=PLANE('',#24676);
#1804=PLANE('',#24677);
#1805=PLANE('',#24679);
#1806=PLANE('',#24680);
#1807=PLANE('',#24682);
#1808=PLANE('',#24683);
#1809=PLANE('',#24685);
#1810=PLANE('',#24686);
#1811=PLANE('',#24688);
#1812=PLANE('',#24689);
#1813=PLANE('',#24691);
#1814=PLANE('',#24692);
#1815=PLANE('',#24694);
#1816=PLANE('',#24695);
#1817=PLANE('',#24697);
#1818=PLANE('',#24698);
#1819=PLANE('',#24700);
#1820=PLANE('',#24701);
#1821=PLANE('',#24703);
#1822=PLANE('',#24704);
#1823=PLANE('',#24707);
#1824=PLANE('',#24708);
#1825=PLANE('',#24711);
#1826=PLANE('',#24712);
#1827=PLANE('',#24714);
#1828=PLANE('',#24715);
#1829=PLANE('',#24717);
#1830=PLANE('',#24718);
#1831=PLANE('',#24720);
#1832=PLANE('',#24721);
#1833=PLANE('',#24723);
#1834=PLANE('',#24724);
#1835=PLANE('',#24726);
#1836=PLANE('',#24727);
#1837=PLANE('',#24729);
#1838=PLANE('',#24730);
#1839=PLANE('',#24732);
#1840=PLANE('',#24733);
#1841=PLANE('',#24735);
#1842=PLANE('',#24736);
#1843=PLANE('',#24738);
#1844=PLANE('',#24739);
#1845=PLANE('',#24741);
#1846=PLANE('',#24742);
#1847=PLANE('',#24744);
#1848=PLANE('',#24745);
#1849=PLANE('',#24747);
#1850=PLANE('',#24748);
#1851=PLANE('',#24750);
#1852=PLANE('',#24751);
#1853=PLANE('',#24753);
#1854=PLANE('',#24754);
#1855=PLANE('',#24756);
#1856=PLANE('',#24757);
#1857=PLANE('',#24759);
#1858=PLANE('',#24760);
#1859=PLANE('',#24762);
#1860=PLANE('',#24763);
#1861=PLANE('',#24765);
#1862=PLANE('',#24766);
#1863=PLANE('',#24768);
#1864=PLANE('',#24769);
#1865=PLANE('',#24771);
#1866=PLANE('',#24772);
#1867=PLANE('',#24774);
#1868=PLANE('',#24775);
#1869=PLANE('',#24777);
#1870=PLANE('',#24778);
#1871=PLANE('',#24780);
#1872=PLANE('',#24781);
#1873=PLANE('',#24783);
#1874=PLANE('',#24786);
#1875=PLANE('',#24794);
#2856=FACE_OUTER_BOUND('',#4321,.T.);
#2857=FACE_OUTER_BOUND('',#4322,.T.);
#2858=FACE_OUTER_BOUND('',#4323,.T.);
#2859=FACE_OUTER_BOUND('',#4324,.T.);
#2860=FACE_OUTER_BOUND('',#4325,.T.);
#2861=FACE_OUTER_BOUND('',#4326,.T.);
#2862=FACE_OUTER_BOUND('',#4327,.T.);
#2863=FACE_OUTER_BOUND('',#4328,.T.);
#2864=FACE_OUTER_BOUND('',#4329,.T.);
#2865=FACE_OUTER_BOUND('',#4330,.T.);
#2866=FACE_OUTER_BOUND('',#4331,.T.);
#2867=FACE_OUTER_BOUND('',#4332,.T.);
#2868=FACE_OUTER_BOUND('',#4333,.T.);
#2869=FACE_OUTER_BOUND('',#4334,.T.);
#2870=FACE_OUTER_BOUND('',#4335,.T.);
#2871=FACE_OUTER_BOUND('',#4336,.T.);
#2872=FACE_OUTER_BOUND('',#4337,.T.);
#2873=FACE_OUTER_BOUND('',#4338,.T.);
#2874=FACE_OUTER_BOUND('',#4339,.T.);
#2875=FACE_OUTER_BOUND('',#4340,.T.);
#2876=FACE_OUTER_BOUND('',#4341,.T.);
#2877=FACE_OUTER_BOUND('',#4342,.T.);
#2878=FACE_OUTER_BOUND('',#4343,.T.);
#2879=FACE_OUTER_BOUND('',#4344,.T.);
#2880=FACE_OUTER_BOUND('',#4345,.T.);
#2881=FACE_OUTER_BOUND('',#4346,.T.);
#2882=FACE_OUTER_BOUND('',#4347,.T.);
#2883=FACE_OUTER_BOUND('',#4348,.T.);
#2884=FACE_OUTER_BOUND('',#4349,.T.);
#2885=FACE_OUTER_BOUND('',#4350,.T.);
#2886=FACE_OUTER_BOUND('',#4351,.T.);
#2887=FACE_OUTER_BOUND('',#4352,.T.);
#2888=FACE_OUTER_BOUND('',#4353,.T.);
#2889=FACE_OUTER_BOUND('',#4354,.T.);
#2890=FACE_OUTER_BOUND('',#4355,.T.);
#2891=FACE_OUTER_BOUND('',#4356,.T.);
#2892=FACE_OUTER_BOUND('',#4357,.T.);
#2893=FACE_OUTER_BOUND('',#4358,.T.);
#2894=FACE_OUTER_BOUND('',#4359,.T.);
#2895=FACE_OUTER_BOUND('',#4360,.T.);
#2896=FACE_OUTER_BOUND('',#4361,.T.);
#2897=FACE_OUTER_BOUND('',#4362,.T.);
#2898=FACE_OUTER_BOUND('',#4363,.T.);
#2899=FACE_OUTER_BOUND('',#4364,.T.);
#2900=FACE_OUTER_BOUND('',#4365,.T.);
#2901=FACE_OUTER_BOUND('',#4366,.T.);
#2902=FACE_OUTER_BOUND('',#4367,.T.);
#2903=FACE_OUTER_BOUND('',#4368,.T.);
#2904=FACE_OUTER_BOUND('',#4369,.T.);
#2905=FACE_OUTER_BOUND('',#4370,.T.);
#2906=FACE_OUTER_BOUND('',#4371,.T.);
#2907=FACE_OUTER_BOUND('',#4372,.T.);
#2908=FACE_OUTER_BOUND('',#4373,.T.);
#2909=FACE_OUTER_BOUND('',#4374,.T.);
#2910=FACE_OUTER_BOUND('',#4375,.T.);
#2911=FACE_OUTER_BOUND('',#4376,.T.);
#2912=FACE_OUTER_BOUND('',#4377,.T.);
#2913=FACE_OUTER_BOUND('',#4378,.T.);
#2914=FACE_OUTER_BOUND('',#4379,.T.);
#2915=FACE_OUTER_BOUND('',#4380,.T.);
#2916=FACE_OUTER_BOUND('',#4381,.T.);
#2917=FACE_OUTER_BOUND('',#4382,.T.);
#2918=FACE_OUTER_BOUND('',#4383,.T.);
#2919=FACE_OUTER_BOUND('',#4384,.T.);
#2920=FACE_OUTER_BOUND('',#4385,.T.);
#2921=FACE_OUTER_BOUND('',#4386,.T.);
#2922=FACE_OUTER_BOUND('',#4387,.T.);
#2923=FACE_OUTER_BOUND('',#4388,.T.);
#2924=FACE_OUTER_BOUND('',#4389,.T.);
#2925=FACE_OUTER_BOUND('',#4390,.T.);
#2926=FACE_OUTER_BOUND('',#4391,.T.);
#2927=FACE_OUTER_BOUND('',#4392,.T.);
#2928=FACE_OUTER_BOUND('',#4393,.T.);
#2929=FACE_OUTER_BOUND('',#4394,.T.);
#2930=FACE_OUTER_BOUND('',#4395,.T.);
#2931=FACE_OUTER_BOUND('',#4396,.T.);
#2932=FACE_OUTER_BOUND('',#4397,.T.);
#2933=FACE_OUTER_BOUND('',#4398,.T.);
#2934=FACE_OUTER_BOUND('',#4399,.T.);
#2935=FACE_OUTER_BOUND('',#4400,.T.);
#2936=FACE_OUTER_BOUND('',#4401,.T.);
#2937=FACE_OUTER_BOUND('',#4402,.T.);
#2938=FACE_OUTER_BOUND('',#4403,.T.);
#2939=FACE_OUTER_BOUND('',#4404,.T.);
#2940=FACE_OUTER_BOUND('',#4405,.T.);
#2941=FACE_OUTER_BOUND('',#4406,.T.);
#2942=FACE_OUTER_BOUND('',#4407,.T.);
#2943=FACE_OUTER_BOUND('',#4408,.T.);
#2944=FACE_OUTER_BOUND('',#4409,.T.);
#2945=FACE_OUTER_BOUND('',#4410,.T.);
#2946=FACE_OUTER_BOUND('',#4411,.T.);
#2947=FACE_OUTER_BOUND('',#4412,.T.);
#2948=FACE_OUTER_BOUND('',#4413,.T.);
#2949=FACE_OUTER_BOUND('',#4414,.T.);
#2950=FACE_OUTER_BOUND('',#4415,.T.);
#2951=FACE_OUTER_BOUND('',#4416,.T.);
#2952=FACE_OUTER_BOUND('',#4417,.T.);
#2953=FACE_OUTER_BOUND('',#4418,.T.);
#2954=FACE_OUTER_BOUND('',#4419,.T.);
#2955=FACE_OUTER_BOUND('',#4420,.T.);
#2956=FACE_OUTER_BOUND('',#4421,.T.);
#2957=FACE_OUTER_BOUND('',#4422,.T.);
#2958=FACE_OUTER_BOUND('',#4423,.T.);
#2959=FACE_OUTER_BOUND('',#4424,.T.);
#2960=FACE_OUTER_BOUND('',#4425,.T.);
#2961=FACE_OUTER_BOUND('',#4426,.T.);
#2962=FACE_OUTER_BOUND('',#4427,.T.);
#2963=FACE_OUTER_BOUND('',#4428,.T.);
#2964=FACE_OUTER_BOUND('',#4429,.T.);
#2965=FACE_OUTER_BOUND('',#4430,.T.);
#2966=FACE_OUTER_BOUND('',#4431,.T.);
#2967=FACE_OUTER_BOUND('',#4432,.T.);
#2968=FACE_OUTER_BOUND('',#4433,.T.);
#2969=FACE_OUTER_BOUND('',#4434,.T.);
#2970=FACE_OUTER_BOUND('',#4435,.T.);
#2971=FACE_OUTER_BOUND('',#4436,.T.);
#2972=FACE_OUTER_BOUND('',#4437,.T.);
#2973=FACE_OUTER_BOUND('',#4438,.T.);
#2974=FACE_OUTER_BOUND('',#4439,.T.);
#2975=FACE_OUTER_BOUND('',#4440,.T.);
#2976=FACE_OUTER_BOUND('',#4441,.T.);
#2977=FACE_OUTER_BOUND('',#4442,.T.);
#2978=FACE_OUTER_BOUND('',#4443,.T.);
#2979=FACE_OUTER_BOUND('',#4444,.T.);
#2980=FACE_OUTER_BOUND('',#4445,.T.);
#2981=FACE_OUTER_BOUND('',#4446,.T.);
#2982=FACE_OUTER_BOUND('',#4447,.T.);
#2983=FACE_OUTER_BOUND('',#4448,.T.);
#2984=FACE_OUTER_BOUND('',#4449,.T.);
#2985=FACE_OUTER_BOUND('',#4450,.T.);
#2986=FACE_OUTER_BOUND('',#4451,.T.);
#2987=FACE_OUTER_BOUND('',#4452,.T.);
#2988=FACE_OUTER_BOUND('',#4453,.T.);
#2989=FACE_OUTER_BOUND('',#4454,.T.);
#2990=FACE_OUTER_BOUND('',#4456,.T.);
#2991=FACE_OUTER_BOUND('',#4457,.T.);
#2992=FACE_OUTER_BOUND('',#4481,.T.);
#2993=FACE_OUTER_BOUND('',#4482,.T.);
#4321=EDGE_LOOP('',(#17797,#17798,#17799,#17800,#17801,#17802,#17803,#17804));
#4322=EDGE_LOOP('',(#17805,#17806,#17807,#17808));
#4323=EDGE_LOOP('',(#17809,#17810,#17811,#17812));
#4324=EDGE_LOOP('',(#17813,#17814,#17815,#17816));
#4325=EDGE_LOOP('',(#17817,#17818,#17819,#17820));
#4326=EDGE_LOOP('',(#17821,#17822,#17823,#17824));
#4327=EDGE_LOOP('',(#17825,#17826,#17827,#17828));
#4328=EDGE_LOOP('',(#17829,#17830,#17831,#17832));
#4329=EDGE_LOOP('',(#17833,#17834,#17835,#17836));
#4330=EDGE_LOOP('',(#17837,#17838,#17839,#17840));
#4331=EDGE_LOOP('',(#17841,#17842,#17843,#17844));
#4332=EDGE_LOOP('',(#17845,#17846,#17847,#17848));
#4333=EDGE_LOOP('',(#17849,#17850,#17851,#17852));
#4334=EDGE_LOOP('',(#17853,#17854,#17855,#17856));
#4335=EDGE_LOOP('',(#17857,#17858,#17859,#17860));
#4336=EDGE_LOOP('',(#17861,#17862,#17863,#17864));
#4337=EDGE_LOOP('',(#17865,#17866,#17867,#17868));
#4338=EDGE_LOOP('',(#17869,#17870,#17871,#17872));
#4339=EDGE_LOOP('',(#17873,#17874,#17875,#17876));
#4340=EDGE_LOOP('',(#17877,#17878,#17879,#17880));
#4341=EDGE_LOOP('',(#17881,#17882,#17883,#17884));
#4342=EDGE_LOOP('',(#17885,#17886,#17887,#17888));
#4343=EDGE_LOOP('',(#17889,#17890,#17891,#17892));
#4344=EDGE_LOOP('',(#17893,#17894,#17895,#17896));
#4345=EDGE_LOOP('',(#17897,#17898,#17899,#17900));
#4346=EDGE_LOOP('',(#17901,#17902,#17903,#17904));
#4347=EDGE_LOOP('',(#17905,#17906,#17907,#17908));
#4348=EDGE_LOOP('',(#17909,#17910,#17911,#17912));
#4349=EDGE_LOOP('',(#17913,#17914,#17915,#17916,#17917));
#4350=EDGE_LOOP('',(#17918,#17919,#17920,#17921,#17922,#17923,#17924,#17925,
#17926,#17927,#17928,#17929,#17930,#17931,#17932,#17933,#17934,#17935,#17936,
#17937,#17938,#17939,#17940,#17941,#17942,#17943,#17944,#17945,#17946,#17947,
#17948,#17949,#17950));
#4351=EDGE_LOOP('',(#17951,#17952,#17953,#17954,#17955,#17956));
#4352=EDGE_LOOP('',(#17957,#17958,#17959));
#4353=EDGE_LOOP('',(#17960,#17961,#17962,#17963,#17964,#17965,#17966,#17967,
#17968,#17969,#17970,#17971,#17972,#17973,#17974,#17975,#17976,#17977,#17978,
#17979,#17980,#17981,#17982,#17983,#17984,#17985,#17986,#17987,#17988,#17989,
#17990,#17991));
#4354=EDGE_LOOP('',(#17992,#17993,#17994,#17995));
#4355=EDGE_LOOP('',(#17996,#17997,#17998));
#4356=EDGE_LOOP('',(#17999,#18000,#18001,#18002));
#4357=EDGE_LOOP('',(#18003,#18004,#18005));
#4358=EDGE_LOOP('',(#18006,#18007,#18008,#18009));
#4359=EDGE_LOOP('',(#18010,#18011,#18012));
#4360=EDGE_LOOP('',(#18013,#18014,#18015,#18016));
#4361=EDGE_LOOP('',(#18017,#18018,#18019));
#4362=EDGE_LOOP('',(#18020,#18021,#18022,#18023));
#4363=EDGE_LOOP('',(#18024,#18025,#18026));
#4364=EDGE_LOOP('',(#18027,#18028,#18029,#18030));
#4365=EDGE_LOOP('',(#18031,#18032,#18033));
#4366=EDGE_LOOP('',(#18034,#18035,#18036,#18037));
#4367=EDGE_LOOP('',(#18038,#18039,#18040));
#4368=EDGE_LOOP('',(#18041,#18042,#18043,#18044));
#4369=EDGE_LOOP('',(#18045,#18046,#18047));
#4370=EDGE_LOOP('',(#18048,#18049,#18050,#18051));
#4371=EDGE_LOOP('',(#18052,#18053,#18054));
#4372=EDGE_LOOP('',(#18055,#18056,#18057,#18058));
#4373=EDGE_LOOP('',(#18059,#18060,#18061));
#4374=EDGE_LOOP('',(#18062,#18063,#18064,#18065));
#4375=EDGE_LOOP('',(#18066,#18067,#18068));
#4376=EDGE_LOOP('',(#18069,#18070,#18071,#18072));
#4377=EDGE_LOOP('',(#18073,#18074,#18075));
#4378=EDGE_LOOP('',(#18076,#18077,#18078,#18079));
#4379=EDGE_LOOP('',(#18080,#18081,#18082));
#4380=EDGE_LOOP('',(#18083,#18084,#18085,#18086));
#4381=EDGE_LOOP('',(#18087,#18088,#18089));
#4382=EDGE_LOOP('',(#18090,#18091,#18092,#18093));
#4383=EDGE_LOOP('',(#18094,#18095,#18096));
#4384=EDGE_LOOP('',(#18097,#18098,#18099,#18100));
#4385=EDGE_LOOP('',(#18101,#18102,#18103));
#4386=EDGE_LOOP('',(#18104,#18105,#18106,#18107));
#4387=EDGE_LOOP('',(#18108,#18109,#18110));
#4388=EDGE_LOOP('',(#18111,#18112,#18113,#18114));
#4389=EDGE_LOOP('',(#18115,#18116,#18117));
#4390=EDGE_LOOP('',(#18118,#18119,#18120,#18121));
#4391=EDGE_LOOP('',(#18122,#18123,#18124));
#4392=EDGE_LOOP('',(#18125,#18126,#18127,#18128));
#4393=EDGE_LOOP('',(#18129,#18130,#18131));
#4394=EDGE_LOOP('',(#18132,#18133,#18134,#18135));
#4395=EDGE_LOOP('',(#18136,#18137,#18138));
#4396=EDGE_LOOP('',(#18139,#18140,#18141,#18142));
#4397=EDGE_LOOP('',(#18143,#18144,#18145));
#4398=EDGE_LOOP('',(#18146,#18147,#18148,#18149));
#4399=EDGE_LOOP('',(#18150,#18151,#18152));
#4400=EDGE_LOOP('',(#18153,#18154,#18155,#18156));
#4401=EDGE_LOOP('',(#18157,#18158,#18159,#18160));
#4402=EDGE_LOOP('',(#18161,#18162,#18163,#18164));
#4403=EDGE_LOOP('',(#18165,#18166,#18167,#18168));
#4404=EDGE_LOOP('',(#18169,#18170,#18171,#18172));
#4405=EDGE_LOOP('',(#18173,#18174,#18175));
#4406=EDGE_LOOP('',(#18176,#18177,#18178,#18179));
#4407=EDGE_LOOP('',(#18180,#18181,#18182));
#4408=EDGE_LOOP('',(#18183,#18184,#18185,#18186));
#4409=EDGE_LOOP('',(#18187,#18188,#18189));
#4410=EDGE_LOOP('',(#18190,#18191,#18192,#18193));
#4411=EDGE_LOOP('',(#18194,#18195,#18196));
#4412=EDGE_LOOP('',(#18197,#18198,#18199,#18200));
#4413=EDGE_LOOP('',(#18201,#18202,#18203));
#4414=EDGE_LOOP('',(#18204,#18205,#18206,#18207));
#4415=EDGE_LOOP('',(#18208,#18209,#18210));
#4416=EDGE_LOOP('',(#18211,#18212,#18213,#18214));
#4417=EDGE_LOOP('',(#18215,#18216,#18217));
#4418=EDGE_LOOP('',(#18218,#18219,#18220,#18221));
#4419=EDGE_LOOP('',(#18222,#18223,#18224));
#4420=EDGE_LOOP('',(#18225,#18226,#18227,#18228));
#4421=EDGE_LOOP('',(#18229,#18230,#18231));
#4422=EDGE_LOOP('',(#18232,#18233,#18234,#18235));
#4423=EDGE_LOOP('',(#18236,#18237,#18238));
#4424=EDGE_LOOP('',(#18239,#18240,#18241,#18242));
#4425=EDGE_LOOP('',(#18243,#18244,#18245));
#4426=EDGE_LOOP('',(#18246,#18247,#18248,#18249));
#4427=EDGE_LOOP('',(#18250,#18251,#18252));
#4428=EDGE_LOOP('',(#18253,#18254,#18255,#18256));
#4429=EDGE_LOOP('',(#18257,#18258,#18259));
#4430=EDGE_LOOP('',(#18260,#18261,#18262,#18263));
#4431=EDGE_LOOP('',(#18264,#18265,#18266));
#4432=EDGE_LOOP('',(#18267,#18268,#18269,#18270));
#4433=EDGE_LOOP('',(#18271,#18272,#18273));
#4434=EDGE_LOOP('',(#18274,#18275,#18276,#18277));
#4435=EDGE_LOOP('',(#18278,#18279,#18280));
#4436=EDGE_LOOP('',(#18281,#18282,#18283,#18284));
#4437=EDGE_LOOP('',(#18285,#18286,#18287));
#4438=EDGE_LOOP('',(#18288,#18289,#18290,#18291));
#4439=EDGE_LOOP('',(#18292,#18293,#18294));
#4440=EDGE_LOOP('',(#18295,#18296,#18297,#18298));
#4441=EDGE_LOOP('',(#18299,#18300,#18301));
#4442=EDGE_LOOP('',(#18302,#18303,#18304,#18305));
#4443=EDGE_LOOP('',(#18306,#18307,#18308));
#4444=EDGE_LOOP('',(#18309,#18310,#18311,#18312));
#4445=EDGE_LOOP('',(#18313,#18314,#18315));
#4446=EDGE_LOOP('',(#18316,#18317,#18318,#18319));
#4447=EDGE_LOOP('',(#18320,#18321,#18322));
#4448=EDGE_LOOP('',(#18323,#18324,#18325,#18326));
#4449=EDGE_LOOP('',(#18327,#18328,#18329));
#4450=EDGE_LOOP('',(#18330,#18331,#18332,#18333));
#4451=EDGE_LOOP('',(#18334,#18335,#18336));
#4452=EDGE_LOOP('',(#18337));
#4453=EDGE_LOOP('',(#18338,#18339,#18340,#18341));
#4454=EDGE_LOOP('',(#18342));
#4455=EDGE_LOOP('',(#18343,#18344,#18345,#18346));
#4456=EDGE_LOOP('',(#18347,#18348,#18349,#18350));
#4457=EDGE_LOOP('',(#18351,#18352,#18353,#18354,#18355,#18356,#18357,#18358,
#18359,#18360,#18361,#18362));
#4458=EDGE_LOOP('',(#18363,#18364,#18365,#18366));
#4459=EDGE_LOOP('',(#18367,#18368,#18369,#18370));
#4460=EDGE_LOOP('',(#18371,#18372,#18373,#18374));
#4461=EDGE_LOOP('',(#18375,#18376,#18377,#18378));
#4462=EDGE_LOOP('',(#18379,#18380,#18381,#18382));
#4463=EDGE_LOOP('',(#18383,#18384,#18385,#18386));
#4464=EDGE_LOOP('',(#18387,#18388,#18389,#18390));
#4465=EDGE_LOOP('',(#18391,#18392,#18393,#18394));
#4466=EDGE_LOOP('',(#18395,#18396,#18397,#18398));
#4467=EDGE_LOOP('',(#18399,#18400,#18401,#18402));
#4468=EDGE_LOOP('',(#18403,#18404,#18405,#18406));
#4469=EDGE_LOOP('',(#18407,#18408,#18409,#18410));
#4470=EDGE_LOOP('',(#18411,#18412,#18413,#18414));
#4471=EDGE_LOOP('',(#18415,#18416,#18417,#18418));
#4472=EDGE_LOOP('',(#18419,#18420,#18421,#18422));
#4473=EDGE_LOOP('',(#18423,#18424,#18425,#18426));
#4474=EDGE_LOOP('',(#18427,#18428,#18429,#18430));
#4475=EDGE_LOOP('',(#18431,#18432,#18433,#18434));
#4476=EDGE_LOOP('',(#18435,#18436,#18437,#18438));
#4477=EDGE_LOOP('',(#18439,#18440,#18441,#18442));
#4478=EDGE_LOOP('',(#18443,#18444,#18445,#18446));
#4479=EDGE_LOOP('',(#18447,#18448,#18449,#18450));
#4480=EDGE_LOOP('',(#18451,#18452,#18453,#18454));
#4481=EDGE_LOOP('',(#18455,#18456,#18457,#18458));
#4482=EDGE_LOOP('',(#18459));
#4483=EDGE_LOOP('',(#18460));
#5531=CIRCLE('',#24597,0.1954);
#5532=CIRCLE('',#24598,0.1954);
#5533=CIRCLE('',#24599,0.1954);
#5534=CIRCLE('',#24614,0.15555);
#5535=CIRCLE('',#24629,0.15555);
#5536=CIRCLE('',#24631,0.15555);
#5537=CIRCLE('',#24634,0.1954);
#5538=CIRCLE('',#24636,0.2);
#5539=CIRCLE('',#24639,0.6);
#5540=CIRCLE('',#24642,0.6);
#5541=CIRCLE('',#24645,0.6);
#5542=CIRCLE('',#24648,0.6);
#5543=CIRCLE('',#24651,0.6);
#5544=CIRCLE('',#24654,0.6);
#5545=CIRCLE('',#24657,0.6);
#5546=CIRCLE('',#24660,0.6);
#5547=CIRCLE('',#24663,0.6);
#5548=CIRCLE('',#24666,0.6);
#5549=CIRCLE('',#24669,0.6);
#5550=CIRCLE('',#24672,0.6);
#5551=CIRCLE('',#24675,0.6);
#5552=CIRCLE('',#24678,0.6);
#5553=CIRCLE('',#24681,0.6);
#5554=CIRCLE('',#24684,0.6);
#5555=CIRCLE('',#24687,0.6);
#5556=CIRCLE('',#24690,0.6);
#5557=CIRCLE('',#24693,0.6);
#5558=CIRCLE('',#24696,0.6);
#5559=CIRCLE('',#24699,0.6);
#5560=CIRCLE('',#24702,0.6);
#5561=CIRCLE('',#24705,0.6);
#5562=CIRCLE('',#24706,0.6);
#5563=CIRCLE('',#24709,0.6);
#5564=CIRCLE('',#24710,0.6);
#5565=CIRCLE('',#24713,0.6);
#5566=CIRCLE('',#24716,0.6);
#5567=CIRCLE('',#24719,0.6);
#5568=CIRCLE('',#24722,0.6);
#5569=CIRCLE('',#24725,0.6);
#5570=CIRCLE('',#24728,0.6);
#5571=CIRCLE('',#24731,0.6);
#5572=CIRCLE('',#24734,0.6);
#5573=CIRCLE('',#24737,0.6);
#5574=CIRCLE('',#24740,0.6);
#5575=CIRCLE('',#24743,0.6);
#5576=CIRCLE('',#24746,0.6);
#5577=CIRCLE('',#24749,0.6);
#5578=CIRCLE('',#24752,0.6);
#5579=CIRCLE('',#24755,0.6);
#5580=CIRCLE('',#24758,0.6);
#5581=CIRCLE('',#24761,0.6);
#5582=CIRCLE('',#24764,0.6);
#5583=CIRCLE('',#24767,0.6);
#5584=CIRCLE('',#24770,0.6);
#5585=CIRCLE('',#24773,0.6);
#5586=CIRCLE('',#24776,0.6);
#5587=CIRCLE('',#24779,0.6);
#5588=CIRCLE('',#24782,0.6);
#5589=CIRCLE('',#24784,0.16);
#5590=CIRCLE('',#24787,0.55);
#5591=CIRCLE('',#24789,0.6);
#5592=CIRCLE('',#24791,0.6);
#5593=CIRCLE('',#24793,0.5);
#6698=LINE('',#36160,#8543);
#6699=LINE('',#36178,#8544);
#6700=LINE('',#36195,#8545);
#6701=LINE('',#36243,#8546);
#6702=LINE('',#36297,#8547);
#6703=LINE('',#36345,#8548);
#6704=LINE('',#36393,#8549);
#6705=LINE('',#36441,#8550);
#6706=LINE('',#36495,#8551);
#6707=LINE('',#36543,#8552);
#6708=LINE('',#36591,#8553);
#6709=LINE('',#36645,#8554);
#6710=LINE('',#36693,#8555);
#6711=LINE('',#36741,#8556);
#6712=LINE('',#36795,#8557);
#6713=LINE('',#36843,#8558);
#6714=LINE('',#36861,#8559);
#6715=LINE('',#36885,#8560);
#6716=LINE('',#36910,#8561);
#6717=LINE('',#36935,#8562);
#6718=LINE('',#36959,#8563);
#6719=LINE('',#36984,#8564);
#6720=LINE('',#37009,#8565);
#6721=LINE('',#37033,#8566);
#6722=LINE('',#37058,#8567);
#6723=LINE('',#37083,#8568);
#6724=LINE('',#37107,#8569);
#6725=LINE('',#37131,#8570);
#6726=LINE('',#37156,#8571);
#6727=LINE('',#37181,#8572);
#6728=LINE('',#38221,#8573);
#6729=LINE('',#38226,#8574);
#6730=LINE('',#38228,#8575);
#6731=LINE('',#38230,#8576);
#6732=LINE('',#38231,#8577);
#6733=LINE('',#38235,#8578);
#6734=LINE('',#38238,#8579);
#6735=LINE('',#38239,#8580);
#6736=LINE('',#38245,#8581);
#6737=LINE('',#38247,#8582);
#6738=LINE('',#38249,#8583);
#6739=LINE('',#38250,#8584);
#6740=LINE('',#38254,#8585);
#6741=LINE('',#38257,#8586);
#6742=LINE('',#38258,#8587);
#6743=LINE('',#38264,#8588);
#6744=LINE('',#38266,#8589);
#6745=LINE('',#38268,#8590);
#6746=LINE('',#38269,#8591);
#6747=LINE('',#38273,#8592);
#6748=LINE('',#38276,#8593);
#6749=LINE('',#38277,#8594);
#6750=LINE('',#38283,#8595);
#6751=LINE('',#38285,#8596);
#6752=LINE('',#38287,#8597);
#6753=LINE('',#38288,#8598);
#6754=LINE('',#38292,#8599);
#6755=LINE('',#38295,#8600);
#6756=LINE('',#38296,#8601);
#6757=LINE('',#38302,#8602);
#6758=LINE('',#38304,#8603);
#6759=LINE('',#38306,#8604);
#6760=LINE('',#38307,#8605);
#6761=LINE('',#38311,#8606);
#6762=LINE('',#38314,#8607);
#6763=LINE('',#38315,#8608);
#6764=LINE('',#38321,#8609);
#6765=LINE('',#38323,#8610);
#6766=LINE('',#38325,#8611);
#6767=LINE('',#38326,#8612);
#6768=LINE('',#38330,#8613);
#6769=LINE('',#38333,#8614);
#6770=LINE('',#38334,#8615);
#6771=LINE('',#38340,#8616);
#6772=LINE('',#38342,#8617);
#6773=LINE('',#38344,#8618);
#6774=LINE('',#38345,#8619);
#6775=LINE('',#38349,#8620);
#6776=LINE('',#38352,#8621);
#6777=LINE('',#38353,#8622);
#6778=LINE('',#38359,#8623);
#6779=LINE('',#38361,#8624);
#6780=LINE('',#38363,#8625);
#6781=LINE('',#38364,#8626);
#6782=LINE('',#38368,#8627);
#6783=LINE('',#38371,#8628);
#6784=LINE('',#38372,#8629);
#6785=LINE('',#38378,#8630);
#6786=LINE('',#38380,#8631);
#6787=LINE('',#38382,#8632);
#6788=LINE('',#38383,#8633);
#6789=LINE('',#38387,#8634);
#6790=LINE('',#38390,#8635);
#6791=LINE('',#38391,#8636);
#6792=LINE('',#38397,#8637);
#6793=LINE('',#38399,#8638);
#6794=LINE('',#38401,#8639);
#6795=LINE('',#38402,#8640);
#6796=LINE('',#38406,#8641);
#6797=LINE('',#38409,#8642);
#6798=LINE('',#38410,#8643);
#6799=LINE('',#38416,#8644);
#6800=LINE('',#38418,#8645);
#6801=LINE('',#38420,#8646);
#6802=LINE('',#38421,#8647);
#6803=LINE('',#38425,#8648);
#6804=LINE('',#38428,#8649);
#6805=LINE('',#38429,#8650);
#6806=LINE('',#38435,#8651);
#6807=LINE('',#38437,#8652);
#6808=LINE('',#38439,#8653);
#6809=LINE('',#38440,#8654);
#6810=LINE('',#38445,#8655);
#6811=LINE('',#38449,#8656);
#6812=LINE('',#38450,#8657);
#6813=LINE('',#38458,#8658);
#6814=LINE('',#38460,#8659);
#6815=LINE('',#38462,#8660);
#6816=LINE('',#38463,#8661);
#6817=LINE('',#38467,#8662);
#6818=LINE('',#38470,#8663);
#6819=LINE('',#38471,#8664);
#6820=LINE('',#38477,#8665);
#6821=LINE('',#38479,#8666);
#6822=LINE('',#38481,#8667);
#6823=LINE('',#38482,#8668);
#6824=LINE('',#38486,#8669);
#6825=LINE('',#38489,#8670);
#6826=LINE('',#38490,#8671);
#6827=LINE('',#38496,#8672);
#6828=LINE('',#38498,#8673);
#6829=LINE('',#38500,#8674);
#6830=LINE('',#38501,#8675);
#6831=LINE('',#38505,#8676);
#6832=LINE('',#38508,#8677);
#6833=LINE('',#38509,#8678);
#6834=LINE('',#38515,#8679);
#6835=LINE('',#38517,#8680);
#6836=LINE('',#38519,#8681);
#6837=LINE('',#38520,#8682);
#6838=LINE('',#38524,#8683);
#6839=LINE('',#38527,#8684);
#6840=LINE('',#38528,#8685);
#6841=LINE('',#38534,#8686);
#6842=LINE('',#38536,#8687);
#6843=LINE('',#38538,#8688);
#6844=LINE('',#38539,#8689);
#6845=LINE('',#38543,#8690);
#6846=LINE('',#38546,#8691);
#6847=LINE('',#38547,#8692);
#6848=LINE('',#38553,#8693);
#6849=LINE('',#38555,#8694);
#6850=LINE('',#38557,#8695);
#6851=LINE('',#38558,#8696);
#6852=LINE('',#38562,#8697);
#6853=LINE('',#38565,#8698);
#6854=LINE('',#38566,#8699);
#6855=LINE('',#38572,#8700);
#6856=LINE('',#38574,#8701);
#6857=LINE('',#38576,#8702);
#6858=LINE('',#38577,#8703);
#6859=LINE('',#38581,#8704);
#6860=LINE('',#38584,#8705);
#6861=LINE('',#38585,#8706);
#6862=LINE('',#38591,#8707);
#6863=LINE('',#38593,#8708);
#6864=LINE('',#38595,#8709);
#6865=LINE('',#38596,#8710);
#6866=LINE('',#38600,#8711);
#6867=LINE('',#38603,#8712);
#6868=LINE('',#38604,#8713);
#6869=LINE('',#38610,#8714);
#6870=LINE('',#38612,#8715);
#6871=LINE('',#38614,#8716);
#6872=LINE('',#38615,#8717);
#6873=LINE('',#38619,#8718);
#6874=LINE('',#38622,#8719);
#6875=LINE('',#38623,#8720);
#6876=LINE('',#38629,#8721);
#6877=LINE('',#38631,#8722);
#6878=LINE('',#38633,#8723);
#6879=LINE('',#38634,#8724);
#6880=LINE('',#38638,#8725);
#6881=LINE('',#38641,#8726);
#6882=LINE('',#38642,#8727);
#6883=LINE('',#38648,#8728);
#6884=LINE('',#38650,#8729);
#6885=LINE('',#38652,#8730);
#6886=LINE('',#38653,#8731);
#6887=LINE('',#38657,#8732);
#6888=LINE('',#38660,#8733);
#6889=LINE('',#38661,#8734);
#6890=LINE('',#38667,#8735);
#6891=LINE('',#38669,#8736);
#6892=LINE('',#38671,#8737);
#6893=LINE('',#38672,#8738);
#6894=LINE('',#38676,#8739);
#6895=LINE('',#38679,#8740);
#6896=LINE('',#38680,#8741);
#6897=LINE('',#38687,#8742);
#6898=LINE('',#38694,#8743);
#6899=LINE('',#38698,#8744);
#6900=LINE('',#38699,#8745);
#6901=LINE('',#38703,#8746);
#8543=VECTOR('',#28702,0.2);
#8544=VECTOR('',#28705,0.2);
#8545=VECTOR('',#28712,0.2);
#8546=VECTOR('',#28715,0.2);
#8547=VECTOR('',#28718,0.2);
#8548=VECTOR('',#28721,0.2);
#8549=VECTOR('',#28724,0.2);
#8550=VECTOR('',#28727,0.2);
#8551=VECTOR('',#28730,0.2);
#8552=VECTOR('',#28733,0.2);
#8553=VECTOR('',#28736,0.2);
#8554=VECTOR('',#28739,0.2);
#8555=VECTOR('',#28742,0.2);
#8556=VECTOR('',#28745,0.2);
#8557=VECTOR('',#28748,0.2);
#8558=VECTOR('',#28751,0.15555);
#8559=VECTOR('',#28756,0.15555);
#8560=VECTOR('',#28759,0.15555);
#8561=VECTOR('',#28762,0.15555);
#8562=VECTOR('',#28765,0.15555);
#8563=VECTOR('',#28768,0.15555);
#8564=VECTOR('',#28771,0.15555);
#8565=VECTOR('',#28774,0.15555);
#8566=VECTOR('',#28777,0.15555);
#8567=VECTOR('',#28780,0.15555);
#8568=VECTOR('',#28783,0.15555);
#8569=VECTOR('',#28786,0.15555);
#8570=VECTOR('',#28789,0.15555);
#8571=VECTOR('',#28792,0.15555);
#8572=VECTOR('',#28795,0.15555);
#8573=VECTOR('',#28810,0.1);
#8574=VECTOR('',#28815,1.);
#8575=VECTOR('',#28816,1.);
#8576=VECTOR('',#28817,1.);
#8577=VECTOR('',#28818,1.);
#8578=VECTOR('',#28823,1.);
#8579=VECTOR('',#28826,1.);
#8580=VECTOR('',#28827,1.);
#8581=VECTOR('',#28834,1.);
#8582=VECTOR('',#28835,1.);
#8583=VECTOR('',#28836,1.);
#8584=VECTOR('',#28837,1.);
#8585=VECTOR('',#28842,1.);
#8586=VECTOR('',#28845,1.);
#8587=VECTOR('',#28846,1.);
#8588=VECTOR('',#28853,1.);
#8589=VECTOR('',#28854,1.);
#8590=VECTOR('',#28855,1.);
#8591=VECTOR('',#28856,1.);
#8592=VECTOR('',#28861,1.);
#8593=VECTOR('',#28864,1.);
#8594=VECTOR('',#28865,1.);
#8595=VECTOR('',#28872,1.);
#8596=VECTOR('',#28873,1.);
#8597=VECTOR('',#28874,1.);
#8598=VECTOR('',#28875,1.);
#8599=VECTOR('',#28880,1.);
#8600=VECTOR('',#28883,1.);
#8601=VECTOR('',#28884,1.);
#8602=VECTOR('',#28891,1.);
#8603=VECTOR('',#28892,1.);
#8604=VECTOR('',#28893,1.);
#8605=VECTOR('',#28894,1.);
#8606=VECTOR('',#28899,1.);
#8607=VECTOR('',#28902,1.);
#8608=VECTOR('',#28903,1.);
#8609=VECTOR('',#28910,1.);
#8610=VECTOR('',#28911,1.);
#8611=VECTOR('',#28912,1.);
#8612=VECTOR('',#28913,1.);
#8613=VECTOR('',#28918,1.);
#8614=VECTOR('',#28921,1.);
#8615=VECTOR('',#28922,1.);
#8616=VECTOR('',#28929,1.);
#8617=VECTOR('',#28930,1.);
#8618=VECTOR('',#28931,1.);
#8619=VECTOR('',#28932,1.);
#8620=VECTOR('',#28937,1.);
#8621=VECTOR('',#28940,1.);
#8622=VECTOR('',#28941,1.);
#8623=VECTOR('',#28948,1.);
#8624=VECTOR('',#28949,1.);
#8625=VECTOR('',#28950,1.);
#8626=VECTOR('',#28951,1.);
#8627=VECTOR('',#28956,1.);
#8628=VECTOR('',#28959,1.);
#8629=VECTOR('',#28960,1.);
#8630=VECTOR('',#28967,1.);
#8631=VECTOR('',#28968,1.);
#8632=VECTOR('',#28969,1.);
#8633=VECTOR('',#28970,1.);
#8634=VECTOR('',#28975,1.);
#8635=VECTOR('',#28978,1.);
#8636=VECTOR('',#28979,1.);
#8637=VECTOR('',#28986,1.);
#8638=VECTOR('',#28987,1.);
#8639=VECTOR('',#28988,1.);
#8640=VECTOR('',#28989,1.);
#8641=VECTOR('',#28994,1.);
#8642=VECTOR('',#28997,1.);
#8643=VECTOR('',#28998,1.);
#8644=VECTOR('',#29005,1.);
#8645=VECTOR('',#29006,1.);
#8646=VECTOR('',#29007,1.);
#8647=VECTOR('',#29008,1.);
#8648=VECTOR('',#29013,1.);
#8649=VECTOR('',#29016,1.);
#8650=VECTOR('',#29017,1.);
#8651=VECTOR('',#29024,1.);
#8652=VECTOR('',#29025,1.);
#8653=VECTOR('',#29026,1.);
#8654=VECTOR('',#29027,1.);
#8655=VECTOR('',#29032,1.);
#8656=VECTOR('',#29037,1.);
#8657=VECTOR('',#29038,1.);
#8658=VECTOR('',#29047,1.);
#8659=VECTOR('',#29048,1.);
#8660=VECTOR('',#29049,1.);
#8661=VECTOR('',#29050,1.);
#8662=VECTOR('',#29055,1.);
#8663=VECTOR('',#29058,1.);
#8664=VECTOR('',#29059,1.);
#8665=VECTOR('',#29066,1.);
#8666=VECTOR('',#29067,1.);
#8667=VECTOR('',#29068,1.);
#8668=VECTOR('',#29069,1.);
#8669=VECTOR('',#29074,1.);
#8670=VECTOR('',#29077,1.);
#8671=VECTOR('',#29078,1.);
#8672=VECTOR('',#29085,1.);
#8673=VECTOR('',#29086,1.);
#8674=VECTOR('',#29087,1.);
#8675=VECTOR('',#29088,1.);
#8676=VECTOR('',#29093,1.);
#8677=VECTOR('',#29096,1.);
#8678=VECTOR('',#29097,1.);
#8679=VECTOR('',#29104,1.);
#8680=VECTOR('',#29105,1.);
#8681=VECTOR('',#29106,1.);
#8682=VECTOR('',#29107,1.);
#8683=VECTOR('',#29112,1.);
#8684=VECTOR('',#29115,1.);
#8685=VECTOR('',#29116,1.);
#8686=VECTOR('',#29123,1.);
#8687=VECTOR('',#29124,1.);
#8688=VECTOR('',#29125,1.);
#8689=VECTOR('',#29126,1.);
#8690=VECTOR('',#29131,1.);
#8691=VECTOR('',#29134,1.);
#8692=VECTOR('',#29135,1.);
#8693=VECTOR('',#29142,1.);
#8694=VECTOR('',#29143,1.);
#8695=VECTOR('',#29144,1.);
#8696=VECTOR('',#29145,1.);
#8697=VECTOR('',#29150,1.);
#8698=VECTOR('',#29153,1.);
#8699=VECTOR('',#29154,1.);
#8700=VECTOR('',#29161,1.);
#8701=VECTOR('',#29162,1.);
#8702=VECTOR('',#29163,1.);
#8703=VECTOR('',#29164,1.);
#8704=VECTOR('',#29169,1.);
#8705=VECTOR('',#29172,1.);
#8706=VECTOR('',#29173,1.);
#8707=VECTOR('',#29180,1.);
#8708=VECTOR('',#29181,1.);
#8709=VECTOR('',#29182,1.);
#8710=VECTOR('',#29183,1.);
#8711=VECTOR('',#29188,1.);
#8712=VECTOR('',#29191,1.);
#8713=VECTOR('',#29192,1.);
#8714=VECTOR('',#29199,1.);
#8715=VECTOR('',#29200,1.);
#8716=VECTOR('',#29201,1.);
#8717=VECTOR('',#29202,1.);
#8718=VECTOR('',#29207,1.);
#8719=VECTOR('',#29210,1.);
#8720=VECTOR('',#29211,1.);
#8721=VECTOR('',#29218,1.);
#8722=VECTOR('',#29219,1.);
#8723=VECTOR('',#29220,1.);
#8724=VECTOR('',#29221,1.);
#8725=VECTOR('',#29226,1.);
#8726=VECTOR('',#29229,1.);
#8727=VECTOR('',#29230,1.);
#8728=VECTOR('',#29237,1.);
#8729=VECTOR('',#29238,1.);
#8730=VECTOR('',#29239,1.);
#8731=VECTOR('',#29240,1.);
#8732=VECTOR('',#29245,1.);
#8733=VECTOR('',#29248,1.);
#8734=VECTOR('',#29249,1.);
#8735=VECTOR('',#29256,1.);
#8736=VECTOR('',#29257,1.);
#8737=VECTOR('',#29258,1.);
#8738=VECTOR('',#29259,1.);
#8739=VECTOR('',#29264,1.);
#8740=VECTOR('',#29267,1.);
#8741=VECTOR('',#29268,1.);
#8742=VECTOR('',#29279,0.18);
#8743=VECTOR('',#29288,0.575);
#8744=VECTOR('',#29293,0.6);
#8745=VECTOR('',#29294,0.6);
#8746=VECTOR('',#29299,0.55);
#10386=VERTEX_POINT('',#36158);
#10387=VERTEX_POINT('',#36159);
#10388=VERTEX_POINT('',#36161);
#10389=VERTEX_POINT('',#36175);
#10390=VERTEX_POINT('',#36177);
#10391=VERTEX_POINT('',#36180);
#10392=VERTEX_POINT('',#36193);
#10393=VERTEX_POINT('',#36194);
#10394=VERTEX_POINT('',#36241);
#10395=VERTEX_POINT('',#36242);
#10396=VERTEX_POINT('',#36295);
#10397=VERTEX_POINT('',#36296);
#10398=VERTEX_POINT('',#36343);
#10399=VERTEX_POINT('',#36344);
#10400=VERTEX_POINT('',#36391);
#10401=VERTEX_POINT('',#36392);
#10402=VERTEX_POINT('',#36439);
#10403=VERTEX_POINT('',#36440);
#10404=VERTEX_POINT('',#36493);
#10405=VERTEX_POINT('',#36494);
#10406=VERTEX_POINT('',#36541);
#10407=VERTEX_POINT('',#36542);
#10408=VERTEX_POINT('',#36589);
#10409=VERTEX_POINT('',#36590);
#10410=VERTEX_POINT('',#36643);
#10411=VERTEX_POINT('',#36644);
#10412=VERTEX_POINT('',#36691);
#10413=VERTEX_POINT('',#36692);
#10414=VERTEX_POINT('',#36739);
#10415=VERTEX_POINT('',#36740);
#10416=VERTEX_POINT('',#36793);
#10417=VERTEX_POINT('',#36794);
#10418=VERTEX_POINT('',#36841);
#10419=VERTEX_POINT('',#36842);
#10420=VERTEX_POINT('',#36844);
#10421=VERTEX_POINT('',#36851);
#10422=VERTEX_POINT('',#36859);
#10423=VERTEX_POINT('',#36860);
#10424=VERTEX_POINT('',#36883);
#10425=VERTEX_POINT('',#36884);
#10426=VERTEX_POINT('',#36908);
#10427=VERTEX_POINT('',#36909);
#10428=VERTEX_POINT('',#36933);
#10429=VERTEX_POINT('',#36934);
#10430=VERTEX_POINT('',#36957);
#10431=VERTEX_POINT('',#36958);
#10432=VERTEX_POINT('',#36982);
#10433=VERTEX_POINT('',#36983);
#10434=VERTEX_POINT('',#37007);
#10435=VERTEX_POINT('',#37008);
#10436=VERTEX_POINT('',#37031);
#10437=VERTEX_POINT('',#37032);
#10438=VERTEX_POINT('',#37056);
#10439=VERTEX_POINT('',#37057);
#10440=VERTEX_POINT('',#37081);
#10441=VERTEX_POINT('',#37082);
#10442=VERTEX_POINT('',#37105);
#10443=VERTEX_POINT('',#37106);
#10444=VERTEX_POINT('',#37129);
#10445=VERTEX_POINT('',#37130);
#10446=VERTEX_POINT('',#37154);
#10447=VERTEX_POINT('',#37155);
#10448=VERTEX_POINT('',#37179);
#10449=VERTEX_POINT('',#37180);
#10450=VERTEX_POINT('',#37182);
#10451=VERTEX_POINT('',#37583);
#10452=VERTEX_POINT('',#37655);
#10453=VERTEX_POINT('',#38147);
#10454=VERTEX_POINT('',#38219);
#10455=VERTEX_POINT('',#38220);
#10456=VERTEX_POINT('',#38224);
#10457=VERTEX_POINT('',#38225);
#10458=VERTEX_POINT('',#38227);
#10459=VERTEX_POINT('',#38229);
#10460=VERTEX_POINT('',#38233);
#10461=VERTEX_POINT('',#38237);
#10462=VERTEX_POINT('',#38243);
#10463=VERTEX_POINT('',#38244);
#10464=VERTEX_POINT('',#38246);
#10465=VERTEX_POINT('',#38248);
#10466=VERTEX_POINT('',#38252);
#10467=VERTEX_POINT('',#38256);
#10468=VERTEX_POINT('',#38262);
#10469=VERTEX_POINT('',#38263);
#10470=VERTEX_POINT('',#38265);
#10471=VERTEX_POINT('',#38267);
#10472=VERTEX_POINT('',#38271);
#10473=VERTEX_POINT('',#38275);
#10474=VERTEX_POINT('',#38281);
#10475=VERTEX_POINT('',#38282);
#10476=VERTEX_POINT('',#38284);
#10477=VERTEX_POINT('',#38286);
#10478=VERTEX_POINT('',#38290);
#10479=VERTEX_POINT('',#38294);
#10480=VERTEX_POINT('',#38300);
#10481=VERTEX_POINT('',#38301);
#10482=VERTEX_POINT('',#38303);
#10483=VERTEX_POINT('',#38305);
#10484=VERTEX_POINT('',#38309);
#10485=VERTEX_POINT('',#38313);
#10486=VERTEX_POINT('',#38319);
#10487=VERTEX_POINT('',#38320);
#10488=VERTEX_POINT('',#38322);
#10489=VERTEX_POINT('',#38324);
#10490=VERTEX_POINT('',#38328);
#10491=VERTEX_POINT('',#38332);
#10492=VERTEX_POINT('',#38338);
#10493=VERTEX_POINT('',#38339);
#10494=VERTEX_POINT('',#38341);
#10495=VERTEX_POINT('',#38343);
#10496=VERTEX_POINT('',#38347);
#10497=VERTEX_POINT('',#38351);
#10498=VERTEX_POINT('',#38357);
#10499=VERTEX_POINT('',#38358);
#10500=VERTEX_POINT('',#38360);
#10501=VERTEX_POINT('',#38362);
#10502=VERTEX_POINT('',#38366);
#10503=VERTEX_POINT('',#38370);
#10504=VERTEX_POINT('',#38376);
#10505=VERTEX_POINT('',#38377);
#10506=VERTEX_POINT('',#38379);
#10507=VERTEX_POINT('',#38381);
#10508=VERTEX_POINT('',#38385);
#10509=VERTEX_POINT('',#38389);
#10510=VERTEX_POINT('',#38395);
#10511=VERTEX_POINT('',#38396);
#10512=VERTEX_POINT('',#38398);
#10513=VERTEX_POINT('',#38400);
#10514=VERTEX_POINT('',#38404);
#10515=VERTEX_POINT('',#38408);
#10516=VERTEX_POINT('',#38414);
#10517=VERTEX_POINT('',#38415);
#10518=VERTEX_POINT('',#38417);
#10519=VERTEX_POINT('',#38419);
#10520=VERTEX_POINT('',#38423);
#10521=VERTEX_POINT('',#38427);
#10522=VERTEX_POINT('',#38433);
#10523=VERTEX_POINT('',#38434);
#10524=VERTEX_POINT('',#38436);
#10525=VERTEX_POINT('',#38438);
#10526=VERTEX_POINT('',#38442);
#10527=VERTEX_POINT('',#38444);
#10528=VERTEX_POINT('',#38448);
#10529=VERTEX_POINT('',#38452);
#10530=VERTEX_POINT('',#38456);
#10531=VERTEX_POINT('',#38457);
#10532=VERTEX_POINT('',#38459);
#10533=VERTEX_POINT('',#38461);
#10534=VERTEX_POINT('',#38465);
#10535=VERTEX_POINT('',#38469);
#10536=VERTEX_POINT('',#38475);
#10537=VERTEX_POINT('',#38476);
#10538=VERTEX_POINT('',#38478);
#10539=VERTEX_POINT('',#38480);
#10540=VERTEX_POINT('',#38484);
#10541=VERTEX_POINT('',#38488);
#10542=VERTEX_POINT('',#38494);
#10543=VERTEX_POINT('',#38495);
#10544=VERTEX_POINT('',#38497);
#10545=VERTEX_POINT('',#38499);
#10546=VERTEX_POINT('',#38503);
#10547=VERTEX_POINT('',#38507);
#10548=VERTEX_POINT('',#38513);
#10549=VERTEX_POINT('',#38514);
#10550=VERTEX_POINT('',#38516);
#10551=VERTEX_POINT('',#38518);
#10552=VERTEX_POINT('',#38522);
#10553=VERTEX_POINT('',#38526);
#10554=VERTEX_POINT('',#38532);
#10555=VERTEX_POINT('',#38533);
#10556=VERTEX_POINT('',#38535);
#10557=VERTEX_POINT('',#38537);
#10558=VERTEX_POINT('',#38541);
#10559=VERTEX_POINT('',#38545);
#10560=VERTEX_POINT('',#38551);
#10561=VERTEX_POINT('',#38552);
#10562=VERTEX_POINT('',#38554);
#10563=VERTEX_POINT('',#38556);
#10564=VERTEX_POINT('',#38560);
#10565=VERTEX_POINT('',#38564);
#10566=VERTEX_POINT('',#38570);
#10567=VERTEX_POINT('',#38571);
#10568=VERTEX_POINT('',#38573);
#10569=VERTEX_POINT('',#38575);
#10570=VERTEX_POINT('',#38579);
#10571=VERTEX_POINT('',#38583);
#10572=VERTEX_POINT('',#38589);
#10573=VERTEX_POINT('',#38590);
#10574=VERTEX_POINT('',#38592);
#10575=VERTEX_POINT('',#38594);
#10576=VERTEX_POINT('',#38598);
#10577=VERTEX_POINT('',#38602);
#10578=VERTEX_POINT('',#38608);
#10579=VERTEX_POINT('',#38609);
#10580=VERTEX_POINT('',#38611);
#10581=VERTEX_POINT('',#38613);
#10582=VERTEX_POINT('',#38617);
#10583=VERTEX_POINT('',#38621);
#10584=VERTEX_POINT('',#38627);
#10585=VERTEX_POINT('',#38628);
#10586=VERTEX_POINT('',#38630);
#10587=VERTEX_POINT('',#38632);
#10588=VERTEX_POINT('',#38636);
#10589=VERTEX_POINT('',#38640);
#10590=VERTEX_POINT('',#38646);
#10591=VERTEX_POINT('',#38647);
#10592=VERTEX_POINT('',#38649);
#10593=VERTEX_POINT('',#38651);
#10594=VERTEX_POINT('',#38655);
#10595=VERTEX_POINT('',#38659);
#10596=VERTEX_POINT('',#38665);
#10597=VERTEX_POINT('',#38666);
#10598=VERTEX_POINT('',#38668);
#10599=VERTEX_POINT('',#38670);
#10600=VERTEX_POINT('',#38674);
#10601=VERTEX_POINT('',#38678);
#10602=VERTEX_POINT('',#38684);
#10603=VERTEX_POINT('',#38689);
#10604=VERTEX_POINT('',#38692);
#10605=VERTEX_POINT('',#38696);
#10606=VERTEX_POINT('',#38701);
#13076=EDGE_CURVE('',#10386,#10387,#6698,.T.);
#13077=EDGE_CURVE('',#10386,#10388,#424,.T.);
#13078=EDGE_CURVE('',#10388,#10389,#5531,.T.);
#13079=EDGE_CURVE('',#10389,#10390,#6699,.T.);
#13080=EDGE_CURVE('',#10390,#10390,#5532,.T.);
#13081=EDGE_CURVE('',#10389,#10391,#5533,.T.);
#13082=EDGE_CURVE('',#10391,#10387,#425,.T.);
#13083=EDGE_CURVE('',#10392,#10393,#6700,.T.);
#13084=EDGE_CURVE('',#10392,#10386,#426,.T.);
#13085=EDGE_CURVE('',#10387,#10393,#427,.T.);
#13086=EDGE_CURVE('',#10394,#10395,#6701,.T.);
#13087=EDGE_CURVE('',#10394,#10392,#428,.T.);
#13088=EDGE_CURVE('',#10393,#10395,#429,.T.);
#13089=EDGE_CURVE('',#10396,#10397,#6702,.T.);
#13090=EDGE_CURVE('',#10396,#10394,#430,.T.);
#13091=EDGE_CURVE('',#10395,#10397,#431,.T.);
#13092=EDGE_CURVE('',#10398,#10399,#6703,.T.);
#13093=EDGE_CURVE('',#10398,#10396,#432,.T.);
#13094=EDGE_CURVE('',#10397,#10399,#433,.T.);
#13095=EDGE_CURVE('',#10400,#10401,#6704,.T.);
#13096=EDGE_CURVE('',#10400,#10398,#434,.T.);
#13097=EDGE_CURVE('',#10399,#10401,#435,.T.);
#13098=EDGE_CURVE('',#10402,#10403,#6705,.T.);
#13099=EDGE_CURVE('',#10402,#10400,#436,.T.);
#13100=EDGE_CURVE('',#10401,#10403,#437,.T.);
#13101=EDGE_CURVE('',#10404,#10405,#6706,.T.);
#13102=EDGE_CURVE('',#10404,#10402,#438,.T.);
#13103=EDGE_CURVE('',#10403,#10405,#439,.T.);
#13104=EDGE_CURVE('',#10406,#10407,#6707,.T.);
#13105=EDGE_CURVE('',#10406,#10404,#440,.T.);
#13106=EDGE_CURVE('',#10405,#10407,#441,.T.);
#13107=EDGE_CURVE('',#10408,#10409,#6708,.T.);
#13108=EDGE_CURVE('',#10408,#10406,#442,.T.);
#13109=EDGE_CURVE('',#10407,#10409,#443,.T.);
#13110=EDGE_CURVE('',#10410,#10411,#6709,.T.);
#13111=EDGE_CURVE('',#10410,#10408,#444,.T.);
#13112=EDGE_CURVE('',#10409,#10411,#445,.T.);
#13113=EDGE_CURVE('',#10412,#10413,#6710,.T.);
#13114=EDGE_CURVE('',#10412,#10410,#446,.T.);
#13115=EDGE_CURVE('',#10411,#10413,#447,.T.);
#13116=EDGE_CURVE('',#10414,#10415,#6711,.T.);
#13117=EDGE_CURVE('',#10414,#10412,#448,.T.);
#13118=EDGE_CURVE('',#10413,#10415,#449,.T.);
#13119=EDGE_CURVE('',#10416,#10417,#6712,.T.);
#13120=EDGE_CURVE('',#10416,#10414,#450,.T.);
#13121=EDGE_CURVE('',#10415,#10417,#451,.T.);
#13122=EDGE_CURVE('',#10418,#10419,#6713,.T.);
#13123=EDGE_CURVE('',#10418,#10420,#452,.T.);
#13124=EDGE_CURVE('',#10421,#10420,#5534,.T.);
#13125=EDGE_CURVE('',#10419,#10421,#453,.T.);
#13126=EDGE_CURVE('',#10422,#10423,#6714,.T.);
#13127=EDGE_CURVE('',#10422,#10418,#454,.T.);
#13128=EDGE_CURVE('',#10423,#10419,#455,.T.);
#13129=EDGE_CURVE('',#10424,#10425,#6715,.T.);
#13130=EDGE_CURVE('',#10424,#10422,#456,.T.);
#13131=EDGE_CURVE('',#10425,#10423,#457,.T.);
#13132=EDGE_CURVE('',#10426,#10427,#6716,.T.);
#13133=EDGE_CURVE('',#10426,#10424,#458,.T.);
#13134=EDGE_CURVE('',#10427,#10425,#459,.T.);
#13135=EDGE_CURVE('',#10428,#10429,#6717,.T.);
#13136=EDGE_CURVE('',#10428,#10426,#460,.T.);
#13137=EDGE_CURVE('',#10429,#10427,#461,.T.);
#13138=EDGE_CURVE('',#10430,#10431,#6718,.T.);
#13139=EDGE_CURVE('',#10430,#10428,#462,.T.);
#13140=EDGE_CURVE('',#10431,#10429,#463,.T.);
#13141=EDGE_CURVE('',#10432,#10433,#6719,.T.);
#13142=EDGE_CURVE('',#10432,#10430,#464,.T.);
#13143=EDGE_CURVE('',#10433,#10431,#465,.T.);
#13144=EDGE_CURVE('',#10434,#10435,#6720,.T.);
#13145=EDGE_CURVE('',#10434,#10432,#466,.T.);
#13146=EDGE_CURVE('',#10435,#10433,#467,.T.);
#13147=EDGE_CURVE('',#10436,#10437,#6721,.T.);
#13148=EDGE_CURVE('',#10436,#10434,#468,.T.);
#13149=EDGE_CURVE('',#10437,#10435,#469,.T.);
#13150=EDGE_CURVE('',#10438,#10439,#6722,.T.);
#13151=EDGE_CURVE('',#10438,#10436,#470,.T.);
#13152=EDGE_CURVE('',#10439,#10437,#471,.T.);
#13153=EDGE_CURVE('',#10440,#10441,#6723,.T.);
#13154=EDGE_CURVE('',#10440,#10438,#472,.T.);
#13155=EDGE_CURVE('',#10441,#10439,#473,.T.);
#13156=EDGE_CURVE('',#10442,#10443,#6724,.T.);
#13157=EDGE_CURVE('',#10442,#10440,#474,.T.);
#13158=EDGE_CURVE('',#10443,#10441,#475,.T.);
#13159=EDGE_CURVE('',#10444,#10445,#6725,.T.);
#13160=EDGE_CURVE('',#10444,#10442,#476,.T.);
#13161=EDGE_CURVE('',#10445,#10443,#477,.T.);
#13162=EDGE_CURVE('',#10446,#10447,#6726,.T.);
#13163=EDGE_CURVE('',#10446,#10444,#478,.T.);
#13164=EDGE_CURVE('',#10447,#10445,#479,.T.);
#13165=EDGE_CURVE('',#10448,#10449,#6727,.T.);
#13166=EDGE_CURVE('',#10450,#10448,#5535,.T.);
#13167=EDGE_CURVE('',#10450,#10446,#480,.T.);
#13168=EDGE_CURVE('',#10449,#10447,#481,.T.);
#13169=EDGE_CURVE('',#10451,#10421,#482,.T.);
#13170=EDGE_CURVE('',#10417,#10451,#483,.T.);
#13171=EDGE_CURVE('',#10452,#10391,#484,.T.);
#13172=EDGE_CURVE('',#10452,#10449,#485,.T.);
#13173=EDGE_CURVE('',#10388,#10450,#486,.T.);
#13174=EDGE_CURVE('',#10448,#10452,#5536,.T.);
#13175=EDGE_CURVE('',#10420,#10453,#487,.T.);
#13176=EDGE_CURVE('',#10453,#10416,#488,.T.);
#13177=EDGE_CURVE('',#10453,#10451,#5537,.T.);
#13178=EDGE_CURVE('',#10454,#10455,#6728,.T.);
#13179=EDGE_CURVE('',#10455,#10455,#5538,.T.);
#13180=EDGE_CURVE('',#10456,#10457,#6729,.T.);
#13181=EDGE_CURVE('',#10458,#10456,#6730,.T.);
#13182=EDGE_CURVE('',#10458,#10459,#6731,.T.);
#13183=EDGE_CURVE('',#10459,#10457,#6732,.T.);
#13184=EDGE_CURVE('',#10457,#10460,#5539,.T.);
#13185=EDGE_CURVE('',#10460,#10459,#6733,.T.);
#13186=EDGE_CURVE('',#10460,#10461,#6734,.T.);
#13187=EDGE_CURVE('',#10461,#10458,#6735,.T.);
#13188=EDGE_CURVE('',#10461,#10456,#5540,.T.);
#13189=EDGE_CURVE('',#10462,#10463,#6736,.T.);
#13190=EDGE_CURVE('',#10464,#10462,#6737,.T.);
#13191=EDGE_CURVE('',#10464,#10465,#6738,.T.);
#13192=EDGE_CURVE('',#10465,#10463,#6739,.T.);
#13193=EDGE_CURVE('',#10463,#10466,#5541,.T.);
#13194=EDGE_CURVE('',#10466,#10465,#6740,.T.);
#13195=EDGE_CURVE('',#10466,#10467,#6741,.T.);
#13196=EDGE_CURVE('',#10467,#10464,#6742,.T.);
#13197=EDGE_CURVE('',#10467,#10462,#5542,.T.);
#13198=EDGE_CURVE('',#10468,#10469,#6743,.T.);
#13199=EDGE_CURVE('',#10470,#10468,#6744,.T.);
#13200=EDGE_CURVE('',#10470,#10471,#6745,.T.);
#13201=EDGE_CURVE('',#10471,#10469,#6746,.T.);
#13202=EDGE_CURVE('',#10469,#10472,#5543,.T.);
#13203=EDGE_CURVE('',#10472,#10471,#6747,.T.);
#13204=EDGE_CURVE('',#10472,#10473,#6748,.T.);
#13205=EDGE_CURVE('',#10473,#10470,#6749,.T.);
#13206=EDGE_CURVE('',#10473,#10468,#5544,.T.);
#13207=EDGE_CURVE('',#10474,#10475,#6750,.T.);
#13208=EDGE_CURVE('',#10476,#10474,#6751,.T.);
#13209=EDGE_CURVE('',#10476,#10477,#6752,.T.);
#13210=EDGE_CURVE('',#10477,#10475,#6753,.T.);
#13211=EDGE_CURVE('',#10475,#10478,#5545,.T.);
#13212=EDGE_CURVE('',#10478,#10477,#6754,.T.);
#13213=EDGE_CURVE('',#10478,#10479,#6755,.T.);
#13214=EDGE_CURVE('',#10479,#10476,#6756,.T.);
#13215=EDGE_CURVE('',#10479,#10474,#5546,.T.);
#13216=EDGE_CURVE('',#10480,#10481,#6757,.T.);
#13217=EDGE_CURVE('',#10482,#10480,#6758,.T.);
#13218=EDGE_CURVE('',#10482,#10483,#6759,.T.);
#13219=EDGE_CURVE('',#10483,#10481,#6760,.T.);
#13220=EDGE_CURVE('',#10481,#10484,#5547,.T.);
#13221=EDGE_CURVE('',#10484,#10483,#6761,.T.);
#13222=EDGE_CURVE('',#10484,#10485,#6762,.T.);
#13223=EDGE_CURVE('',#10485,#10482,#6763,.T.);
#13224=EDGE_CURVE('',#10485,#10480,#5548,.T.);
#13225=EDGE_CURVE('',#10486,#10487,#6764,.T.);
#13226=EDGE_CURVE('',#10488,#10486,#6765,.T.);
#13227=EDGE_CURVE('',#10488,#10489,#6766,.T.);
#13228=EDGE_CURVE('',#10489,#10487,#6767,.T.);
#13229=EDGE_CURVE('',#10487,#10490,#5549,.T.);
#13230=EDGE_CURVE('',#10490,#10489,#6768,.T.);
#13231=EDGE_CURVE('',#10490,#10491,#6769,.T.);
#13232=EDGE_CURVE('',#10491,#10488,#6770,.T.);
#13233=EDGE_CURVE('',#10491,#10486,#5550,.T.);
#13234=EDGE_CURVE('',#10492,#10493,#6771,.T.);
#13235=EDGE_CURVE('',#10494,#10492,#6772,.T.);
#13236=EDGE_CURVE('',#10494,#10495,#6773,.T.);
#13237=EDGE_CURVE('',#10495,#10493,#6774,.T.);
#13238=EDGE_CURVE('',#10493,#10496,#5551,.T.);
#13239=EDGE_CURVE('',#10496,#10495,#6775,.T.);
#13240=EDGE_CURVE('',#10496,#10497,#6776,.T.);
#13241=EDGE_CURVE('',#10497,#10494,#6777,.T.);
#13242=EDGE_CURVE('',#10497,#10492,#5552,.T.);
#13243=EDGE_CURVE('',#10498,#10499,#6778,.T.);
#13244=EDGE_CURVE('',#10500,#10498,#6779,.T.);
#13245=EDGE_CURVE('',#10500,#10501,#6780,.T.);
#13246=EDGE_CURVE('',#10501,#10499,#6781,.T.);
#13247=EDGE_CURVE('',#10499,#10502,#5553,.T.);
#13248=EDGE_CURVE('',#10502,#10501,#6782,.T.);
#13249=EDGE_CURVE('',#10502,#10503,#6783,.T.);
#13250=EDGE_CURVE('',#10503,#10500,#6784,.T.);
#13251=EDGE_CURVE('',#10503,#10498,#5554,.T.);
#13252=EDGE_CURVE('',#10504,#10505,#6785,.T.);
#13253=EDGE_CURVE('',#10506,#10504,#6786,.T.);
#13254=EDGE_CURVE('',#10506,#10507,#6787,.T.);
#13255=EDGE_CURVE('',#10507,#10505,#6788,.T.);
#13256=EDGE_CURVE('',#10505,#10508,#5555,.T.);
#13257=EDGE_CURVE('',#10508,#10507,#6789,.T.);
#13258=EDGE_CURVE('',#10508,#10509,#6790,.T.);
#13259=EDGE_CURVE('',#10509,#10506,#6791,.T.);
#13260=EDGE_CURVE('',#10509,#10504,#5556,.T.);
#13261=EDGE_CURVE('',#10510,#10511,#6792,.T.);
#13262=EDGE_CURVE('',#10512,#10510,#6793,.T.);
#13263=EDGE_CURVE('',#10512,#10513,#6794,.T.);
#13264=EDGE_CURVE('',#10513,#10511,#6795,.T.);
#13265=EDGE_CURVE('',#10511,#10514,#5557,.T.);
#13266=EDGE_CURVE('',#10514,#10513,#6796,.T.);
#13267=EDGE_CURVE('',#10514,#10515,#6797,.T.);
#13268=EDGE_CURVE('',#10515,#10512,#6798,.T.);
#13269=EDGE_CURVE('',#10515,#10510,#5558,.T.);
#13270=EDGE_CURVE('',#10516,#10517,#6799,.T.);
#13271=EDGE_CURVE('',#10518,#10516,#6800,.T.);
#13272=EDGE_CURVE('',#10518,#10519,#6801,.T.);
#13273=EDGE_CURVE('',#10519,#10517,#6802,.T.);
#13274=EDGE_CURVE('',#10517,#10520,#5559,.T.);
#13275=EDGE_CURVE('',#10520,#10519,#6803,.T.);
#13276=EDGE_CURVE('',#10520,#10521,#6804,.T.);
#13277=EDGE_CURVE('',#10521,#10518,#6805,.T.);
#13278=EDGE_CURVE('',#10521,#10516,#5560,.T.);
#13279=EDGE_CURVE('',#10522,#10523,#6806,.T.);
#13280=EDGE_CURVE('',#10524,#10522,#6807,.T.);
#13281=EDGE_CURVE('',#10524,#10525,#6808,.T.);
#13282=EDGE_CURVE('',#10525,#10523,#6809,.T.);
#13283=EDGE_CURVE('',#10523,#10526,#5561,.T.);
#13284=EDGE_CURVE('',#10527,#10525,#6810,.T.);
#13285=EDGE_CURVE('',#10526,#10527,#5562,.T.);
#13286=EDGE_CURVE('',#10527,#10528,#6811,.T.);
#13287=EDGE_CURVE('',#10528,#10524,#6812,.T.);
#13288=EDGE_CURVE('',#10528,#10529,#5563,.T.);
#13289=EDGE_CURVE('',#10529,#10522,#5564,.T.);
#13290=EDGE_CURVE('',#10530,#10531,#6813,.T.);
#13291=EDGE_CURVE('',#10532,#10530,#6814,.T.);
#13292=EDGE_CURVE('',#10532,#10533,#6815,.T.);
#13293=EDGE_CURVE('',#10533,#10531,#6816,.T.);
#13294=EDGE_CURVE('',#10531,#10534,#5565,.T.);
#13295=EDGE_CURVE('',#10534,#10533,#6817,.T.);
#13296=EDGE_CURVE('',#10534,#10535,#6818,.T.);
#13297=EDGE_CURVE('',#10535,#10532,#6819,.T.);
#13298=EDGE_CURVE('',#10535,#10530,#5566,.T.);
#13299=EDGE_CURVE('',#10536,#10537,#6820,.T.);
#13300=EDGE_CURVE('',#10538,#10536,#6821,.T.);
#13301=EDGE_CURVE('',#10538,#10539,#6822,.T.);
#13302=EDGE_CURVE('',#10539,#10537,#6823,.T.);
#13303=EDGE_CURVE('',#10537,#10540,#5567,.T.);
#13304=EDGE_CURVE('',#10540,#10539,#6824,.T.);
#13305=EDGE_CURVE('',#10540,#10541,#6825,.T.);
#13306=EDGE_CURVE('',#10541,#10538,#6826,.T.);
#13307=EDGE_CURVE('',#10541,#10536,#5568,.T.);
#13308=EDGE_CURVE('',#10542,#10543,#6827,.T.);
#13309=EDGE_CURVE('',#10544,#10542,#6828,.T.);
#13310=EDGE_CURVE('',#10544,#10545,#6829,.T.);
#13311=EDGE_CURVE('',#10545,#10543,#6830,.T.);
#13312=EDGE_CURVE('',#10543,#10546,#5569,.T.);
#13313=EDGE_CURVE('',#10546,#10545,#6831,.T.);
#13314=EDGE_CURVE('',#10546,#10547,#6832,.T.);
#13315=EDGE_CURVE('',#10547,#10544,#6833,.T.);
#13316=EDGE_CURVE('',#10547,#10542,#5570,.T.);
#13317=EDGE_CURVE('',#10548,#10549,#6834,.T.);
#13318=EDGE_CURVE('',#10550,#10548,#6835,.T.);
#13319=EDGE_CURVE('',#10550,#10551,#6836,.T.);
#13320=EDGE_CURVE('',#10551,#10549,#6837,.T.);
#13321=EDGE_CURVE('',#10549,#10552,#5571,.T.);
#13322=EDGE_CURVE('',#10552,#10551,#6838,.T.);
#13323=EDGE_CURVE('',#10552,#10553,#6839,.T.);
#13324=EDGE_CURVE('',#10553,#10550,#6840,.T.);
#13325=EDGE_CURVE('',#10553,#10548,#5572,.T.);
#13326=EDGE_CURVE('',#10554,#10555,#6841,.T.);
#13327=EDGE_CURVE('',#10556,#10554,#6842,.T.);
#13328=EDGE_CURVE('',#10556,#10557,#6843,.T.);
#13329=EDGE_CURVE('',#10557,#10555,#6844,.T.);
#13330=EDGE_CURVE('',#10555,#10558,#5573,.T.);
#13331=EDGE_CURVE('',#10558,#10557,#6845,.T.);
#13332=EDGE_CURVE('',#10558,#10559,#6846,.T.);
#13333=EDGE_CURVE('',#10559,#10556,#6847,.T.);
#13334=EDGE_CURVE('',#10559,#10554,#5574,.T.);
#13335=EDGE_CURVE('',#10560,#10561,#6848,.T.);
#13336=EDGE_CURVE('',#10562,#10560,#6849,.T.);
#13337=EDGE_CURVE('',#10562,#10563,#6850,.T.);
#13338=EDGE_CURVE('',#10563,#10561,#6851,.T.);
#13339=EDGE_CURVE('',#10561,#10564,#5575,.T.);
#13340=EDGE_CURVE('',#10564,#10563,#6852,.T.);
#13341=EDGE_CURVE('',#10564,#10565,#6853,.T.);
#13342=EDGE_CURVE('',#10565,#10562,#6854,.T.);
#13343=EDGE_CURVE('',#10565,#10560,#5576,.T.);
#13344=EDGE_CURVE('',#10566,#10567,#6855,.T.);
#13345=EDGE_CURVE('',#10568,#10566,#6856,.T.);
#13346=EDGE_CURVE('',#10568,#10569,#6857,.T.);
#13347=EDGE_CURVE('',#10569,#10567,#6858,.T.);
#13348=EDGE_CURVE('',#10567,#10570,#5577,.T.);
#13349=EDGE_CURVE('',#10570,#10569,#6859,.T.);
#13350=EDGE_CURVE('',#10570,#10571,#6860,.T.);
#13351=EDGE_CURVE('',#10571,#10568,#6861,.T.);
#13352=EDGE_CURVE('',#10571,#10566,#5578,.T.);
#13353=EDGE_CURVE('',#10572,#10573,#6862,.T.);
#13354=EDGE_CURVE('',#10574,#10572,#6863,.T.);
#13355=EDGE_CURVE('',#10574,#10575,#6864,.T.);
#13356=EDGE_CURVE('',#10575,#10573,#6865,.T.);
#13357=EDGE_CURVE('',#10573,#10576,#5579,.T.);
#13358=EDGE_CURVE('',#10576,#10575,#6866,.T.);
#13359=EDGE_CURVE('',#10576,#10577,#6867,.T.);
#13360=EDGE_CURVE('',#10577,#10574,#6868,.T.);
#13361=EDGE_CURVE('',#10577,#10572,#5580,.T.);
#13362=EDGE_CURVE('',#10578,#10579,#6869,.T.);
#13363=EDGE_CURVE('',#10580,#10578,#6870,.T.);
#13364=EDGE_CURVE('',#10580,#10581,#6871,.T.);
#13365=EDGE_CURVE('',#10581,#10579,#6872,.T.);
#13366=EDGE_CURVE('',#10579,#10582,#5581,.T.);
#13367=EDGE_CURVE('',#10582,#10581,#6873,.T.);
#13368=EDGE_CURVE('',#10582,#10583,#6874,.T.);
#13369=EDGE_CURVE('',#10583,#10580,#6875,.T.);
#13370=EDGE_CURVE('',#10583,#10578,#5582,.T.);
#13371=EDGE_CURVE('',#10584,#10585,#6876,.T.);
#13372=EDGE_CURVE('',#10586,#10584,#6877,.T.);
#13373=EDGE_CURVE('',#10586,#10587,#6878,.T.);
#13374=EDGE_CURVE('',#10587,#10585,#6879,.T.);
#13375=EDGE_CURVE('',#10585,#10588,#5583,.T.);
#13376=EDGE_CURVE('',#10588,#10587,#6880,.T.);
#13377=EDGE_CURVE('',#10588,#10589,#6881,.T.);
#13378=EDGE_CURVE('',#10589,#10586,#6882,.T.);
#13379=EDGE_CURVE('',#10589,#10584,#5584,.T.);
#13380=EDGE_CURVE('',#10590,#10591,#6883,.T.);
#13381=EDGE_CURVE('',#10592,#10590,#6884,.T.);
#13382=EDGE_CURVE('',#10592,#10593,#6885,.T.);
#13383=EDGE_CURVE('',#10593,#10591,#6886,.T.);
#13384=EDGE_CURVE('',#10591,#10594,#5585,.T.);
#13385=EDGE_CURVE('',#10594,#10593,#6887,.T.);
#13386=EDGE_CURVE('',#10594,#10595,#6888,.T.);
#13387=EDGE_CURVE('',#10595,#10592,#6889,.T.);
#13388=EDGE_CURVE('',#10595,#10590,#5586,.T.);
#13389=EDGE_CURVE('',#10596,#10597,#6890,.T.);
#13390=EDGE_CURVE('',#10598,#10596,#6891,.T.);
#13391=EDGE_CURVE('',#10598,#10599,#6892,.T.);
#13392=EDGE_CURVE('',#10599,#10597,#6893,.T.);
#13393=EDGE_CURVE('',#10597,#10600,#5587,.T.);
#13394=EDGE_CURVE('',#10600,#10599,#6894,.T.);
#13395=EDGE_CURVE('',#10600,#10601,#6895,.T.);
#13396=EDGE_CURVE('',#10601,#10598,#6896,.T.);
#13397=EDGE_CURVE('',#10601,#10596,#5588,.T.);
#13398=EDGE_CURVE('',#10602,#10602,#5589,.T.);
#13399=EDGE_CURVE('',#10390,#10602,#6897,.T.);
#13400=EDGE_CURVE('',#10603,#10603,#5590,.T.);
#13401=EDGE_CURVE('',#10604,#10604,#5591,.T.);
#13402=EDGE_CURVE('',#10604,#10603,#6898,.T.);
#13403=EDGE_CURVE('',#10605,#10605,#5592,.T.);
#13404=EDGE_CURVE('',#10605,#10526,#6899,.T.);
#13405=EDGE_CURVE('',#10529,#10604,#6900,.T.);
#13406=EDGE_CURVE('',#10606,#10606,#5593,.T.);
#13407=EDGE_CURVE('',#10606,#10605,#6901,.T.);
#17797=ORIENTED_EDGE('',*,*,#13076,.F.);
#17798=ORIENTED_EDGE('',*,*,#13077,.T.);
#17799=ORIENTED_EDGE('',*,*,#13078,.T.);
#17800=ORIENTED_EDGE('',*,*,#13079,.T.);
#17801=ORIENTED_EDGE('',*,*,#13080,.T.);
#17802=ORIENTED_EDGE('',*,*,#13079,.F.);
#17803=ORIENTED_EDGE('',*,*,#13081,.T.);
#17804=ORIENTED_EDGE('',*,*,#13082,.T.);
#17805=ORIENTED_EDGE('',*,*,#13083,.F.);
#17806=ORIENTED_EDGE('',*,*,#13084,.T.);
#17807=ORIENTED_EDGE('',*,*,#13076,.T.);
#17808=ORIENTED_EDGE('',*,*,#13085,.T.);
#17809=ORIENTED_EDGE('',*,*,#13086,.F.);
#17810=ORIENTED_EDGE('',*,*,#13087,.T.);
#17811=ORIENTED_EDGE('',*,*,#13083,.T.);
#17812=ORIENTED_EDGE('',*,*,#13088,.T.);
#17813=ORIENTED_EDGE('',*,*,#13089,.F.);
#17814=ORIENTED_EDGE('',*,*,#13090,.T.);
#17815=ORIENTED_EDGE('',*,*,#13086,.T.);
#17816=ORIENTED_EDGE('',*,*,#13091,.T.);
#17817=ORIENTED_EDGE('',*,*,#13092,.F.);
#17818=ORIENTED_EDGE('',*,*,#13093,.T.);
#17819=ORIENTED_EDGE('',*,*,#13089,.T.);
#17820=ORIENTED_EDGE('',*,*,#13094,.T.);
#17821=ORIENTED_EDGE('',*,*,#13095,.F.);
#17822=ORIENTED_EDGE('',*,*,#13096,.T.);
#17823=ORIENTED_EDGE('',*,*,#13092,.T.);
#17824=ORIENTED_EDGE('',*,*,#13097,.T.);
#17825=ORIENTED_EDGE('',*,*,#13098,.F.);
#17826=ORIENTED_EDGE('',*,*,#13099,.T.);
#17827=ORIENTED_EDGE('',*,*,#13095,.T.);
#17828=ORIENTED_EDGE('',*,*,#13100,.T.);
#17829=ORIENTED_EDGE('',*,*,#13101,.F.);
#17830=ORIENTED_EDGE('',*,*,#13102,.T.);
#17831=ORIENTED_EDGE('',*,*,#13098,.T.);
#17832=ORIENTED_EDGE('',*,*,#13103,.T.);
#17833=ORIENTED_EDGE('',*,*,#13104,.F.);
#17834=ORIENTED_EDGE('',*,*,#13105,.T.);
#17835=ORIENTED_EDGE('',*,*,#13101,.T.);
#17836=ORIENTED_EDGE('',*,*,#13106,.T.);
#17837=ORIENTED_EDGE('',*,*,#13107,.F.);
#17838=ORIENTED_EDGE('',*,*,#13108,.T.);
#17839=ORIENTED_EDGE('',*,*,#13104,.T.);
#17840=ORIENTED_EDGE('',*,*,#13109,.T.);
#17841=ORIENTED_EDGE('',*,*,#13110,.F.);
#17842=ORIENTED_EDGE('',*,*,#13111,.T.);
#17843=ORIENTED_EDGE('',*,*,#13107,.T.);
#17844=ORIENTED_EDGE('',*,*,#13112,.T.);
#17845=ORIENTED_EDGE('',*,*,#13113,.F.);
#17846=ORIENTED_EDGE('',*,*,#13114,.T.);
#17847=ORIENTED_EDGE('',*,*,#13110,.T.);
#17848=ORIENTED_EDGE('',*,*,#13115,.T.);
#17849=ORIENTED_EDGE('',*,*,#13116,.F.);
#17850=ORIENTED_EDGE('',*,*,#13117,.T.);
#17851=ORIENTED_EDGE('',*,*,#13113,.T.);
#17852=ORIENTED_EDGE('',*,*,#13118,.T.);
#17853=ORIENTED_EDGE('',*,*,#13119,.F.);
#17854=ORIENTED_EDGE('',*,*,#13120,.T.);
#17855=ORIENTED_EDGE('',*,*,#13116,.T.);
#17856=ORIENTED_EDGE('',*,*,#13121,.T.);
#17857=ORIENTED_EDGE('',*,*,#13122,.F.);
#17858=ORIENTED_EDGE('',*,*,#13123,.T.);
#17859=ORIENTED_EDGE('',*,*,#13124,.F.);
#17860=ORIENTED_EDGE('',*,*,#13125,.F.);
#17861=ORIENTED_EDGE('',*,*,#13126,.F.);
#17862=ORIENTED_EDGE('',*,*,#13127,.T.);
#17863=ORIENTED_EDGE('',*,*,#13122,.T.);
#17864=ORIENTED_EDGE('',*,*,#13128,.F.);
#17865=ORIENTED_EDGE('',*,*,#13129,.F.);
#17866=ORIENTED_EDGE('',*,*,#13130,.T.);
#17867=ORIENTED_EDGE('',*,*,#13126,.T.);
#17868=ORIENTED_EDGE('',*,*,#13131,.F.);
#17869=ORIENTED_EDGE('',*,*,#13132,.F.);
#17870=ORIENTED_EDGE('',*,*,#13133,.T.);
#17871=ORIENTED_EDGE('',*,*,#13129,.T.);
#17872=ORIENTED_EDGE('',*,*,#13134,.F.);
#17873=ORIENTED_EDGE('',*,*,#13135,.F.);
#17874=ORIENTED_EDGE('',*,*,#13136,.T.);
#17875=ORIENTED_EDGE('',*,*,#13132,.T.);
#17876=ORIENTED_EDGE('',*,*,#13137,.F.);
#17877=ORIENTED_EDGE('',*,*,#13138,.F.);
#17878=ORIENTED_EDGE('',*,*,#13139,.T.);
#17879=ORIENTED_EDGE('',*,*,#13135,.T.);
#17880=ORIENTED_EDGE('',*,*,#13140,.F.);
#17881=ORIENTED_EDGE('',*,*,#13141,.F.);
#17882=ORIENTED_EDGE('',*,*,#13142,.T.);
#17883=ORIENTED_EDGE('',*,*,#13138,.T.);
#17884=ORIENTED_EDGE('',*,*,#13143,.F.);
#17885=ORIENTED_EDGE('',*,*,#13144,.F.);
#17886=ORIENTED_EDGE('',*,*,#13145,.T.);
#17887=ORIENTED_EDGE('',*,*,#13141,.T.);
#17888=ORIENTED_EDGE('',*,*,#13146,.F.);
#17889=ORIENTED_EDGE('',*,*,#13147,.F.);
#17890=ORIENTED_EDGE('',*,*,#13148,.T.);
#17891=ORIENTED_EDGE('',*,*,#13144,.T.);
#17892=ORIENTED_EDGE('',*,*,#13149,.F.);
#17893=ORIENTED_EDGE('',*,*,#13150,.F.);
#17894=ORIENTED_EDGE('',*,*,#13151,.T.);
#17895=ORIENTED_EDGE('',*,*,#13147,.T.);
#17896=ORIENTED_EDGE('',*,*,#13152,.F.);
#17897=ORIENTED_EDGE('',*,*,#13153,.F.);
#17898=ORIENTED_EDGE('',*,*,#13154,.T.);
#17899=ORIENTED_EDGE('',*,*,#13150,.T.);
#17900=ORIENTED_EDGE('',*,*,#13155,.F.);
#17901=ORIENTED_EDGE('',*,*,#13156,.F.);
#17902=ORIENTED_EDGE('',*,*,#13157,.T.);
#17903=ORIENTED_EDGE('',*,*,#13153,.T.);
#17904=ORIENTED_EDGE('',*,*,#13158,.F.);
#17905=ORIENTED_EDGE('',*,*,#13159,.F.);
#17906=ORIENTED_EDGE('',*,*,#13160,.T.);
#17907=ORIENTED_EDGE('',*,*,#13156,.T.);
#17908=ORIENTED_EDGE('',*,*,#13161,.F.);
#17909=ORIENTED_EDGE('',*,*,#13162,.F.);
#17910=ORIENTED_EDGE('',*,*,#13163,.T.);
#17911=ORIENTED_EDGE('',*,*,#13159,.T.);
#17912=ORIENTED_EDGE('',*,*,#13164,.F.);
#17913=ORIENTED_EDGE('',*,*,#13165,.F.);
#17914=ORIENTED_EDGE('',*,*,#13166,.F.);
#17915=ORIENTED_EDGE('',*,*,#13167,.T.);
#17916=ORIENTED_EDGE('',*,*,#13162,.T.);
#17917=ORIENTED_EDGE('',*,*,#13168,.F.);
#17918=ORIENTED_EDGE('',*,*,#13169,.F.);
#17919=ORIENTED_EDGE('',*,*,#13170,.F.);
#17920=ORIENTED_EDGE('',*,*,#13121,.F.);
#17921=ORIENTED_EDGE('',*,*,#13118,.F.);
#17922=ORIENTED_EDGE('',*,*,#13115,.F.);
#17923=ORIENTED_EDGE('',*,*,#13112,.F.);
#17924=ORIENTED_EDGE('',*,*,#13109,.F.);
#17925=ORIENTED_EDGE('',*,*,#13106,.F.);
#17926=ORIENTED_EDGE('',*,*,#13103,.F.);
#17927=ORIENTED_EDGE('',*,*,#13100,.F.);
#17928=ORIENTED_EDGE('',*,*,#13097,.F.);
#17929=ORIENTED_EDGE('',*,*,#13094,.F.);
#17930=ORIENTED_EDGE('',*,*,#13091,.F.);
#17931=ORIENTED_EDGE('',*,*,#13088,.F.);
#17932=ORIENTED_EDGE('',*,*,#13085,.F.);
#17933=ORIENTED_EDGE('',*,*,#13082,.F.);
#17934=ORIENTED_EDGE('',*,*,#13171,.F.);
#17935=ORIENTED_EDGE('',*,*,#13172,.T.);
#17936=ORIENTED_EDGE('',*,*,#13168,.T.);
#17937=ORIENTED_EDGE('',*,*,#13164,.T.);
#17938=ORIENTED_EDGE('',*,*,#13161,.T.);
#17939=ORIENTED_EDGE('',*,*,#13158,.T.);
#17940=ORIENTED_EDGE('',*,*,#13155,.T.);
#17941=ORIENTED_EDGE('',*,*,#13152,.T.);
#17942=ORIENTED_EDGE('',*,*,#13149,.T.);
#17943=ORIENTED_EDGE('',*,*,#13146,.T.);
#17944=ORIENTED_EDGE('',*,*,#13143,.T.);
#17945=ORIENTED_EDGE('',*,*,#13140,.T.);
#17946=ORIENTED_EDGE('',*,*,#13137,.T.);
#17947=ORIENTED_EDGE('',*,*,#13134,.T.);
#17948=ORIENTED_EDGE('',*,*,#13131,.T.);
#17949=ORIENTED_EDGE('',*,*,#13128,.T.);
#17950=ORIENTED_EDGE('',*,*,#13125,.T.);
#17951=ORIENTED_EDGE('',*,*,#13078,.F.);
#17952=ORIENTED_EDGE('',*,*,#13173,.T.);
#17953=ORIENTED_EDGE('',*,*,#13166,.T.);
#17954=ORIENTED_EDGE('',*,*,#13174,.T.);
#17955=ORIENTED_EDGE('',*,*,#13171,.T.);
#17956=ORIENTED_EDGE('',*,*,#13081,.F.);
#17957=ORIENTED_EDGE('',*,*,#13165,.T.);
#17958=ORIENTED_EDGE('',*,*,#13172,.F.);
#17959=ORIENTED_EDGE('',*,*,#13174,.F.);
#17960=ORIENTED_EDGE('',*,*,#13175,.F.);
#17961=ORIENTED_EDGE('',*,*,#13123,.F.);
#17962=ORIENTED_EDGE('',*,*,#13127,.F.);
#17963=ORIENTED_EDGE('',*,*,#13130,.F.);
#17964=ORIENTED_EDGE('',*,*,#13133,.F.);
#17965=ORIENTED_EDGE('',*,*,#13136,.F.);
#17966=ORIENTED_EDGE('',*,*,#13139,.F.);
#17967=ORIENTED_EDGE('',*,*,#13142,.F.);
#17968=ORIENTED_EDGE('',*,*,#13145,.F.);
#17969=ORIENTED_EDGE('',*,*,#13148,.F.);
#17970=ORIENTED_EDGE('',*,*,#13151,.F.);
#17971=ORIENTED_EDGE('',*,*,#13154,.F.);
#17972=ORIENTED_EDGE('',*,*,#13157,.F.);
#17973=ORIENTED_EDGE('',*,*,#13160,.F.);
#17974=ORIENTED_EDGE('',*,*,#13163,.F.);
#17975=ORIENTED_EDGE('',*,*,#13167,.F.);
#17976=ORIENTED_EDGE('',*,*,#13173,.F.);
#17977=ORIENTED_EDGE('',*,*,#13077,.F.);
#17978=ORIENTED_EDGE('',*,*,#13084,.F.);
#17979=ORIENTED_EDGE('',*,*,#13087,.F.);
#17980=ORIENTED_EDGE('',*,*,#13090,.F.);
#17981=ORIENTED_EDGE('',*,*,#13093,.F.);
#17982=ORIENTED_EDGE('',*,*,#13096,.F.);
#17983=ORIENTED_EDGE('',*,*,#13099,.F.);
#17984=ORIENTED_EDGE('',*,*,#13102,.F.);
#17985=ORIENTED_EDGE('',*,*,#13105,.F.);
#17986=ORIENTED_EDGE('',*,*,#13108,.F.);
#17987=ORIENTED_EDGE('',*,*,#13111,.F.);
#17988=ORIENTED_EDGE('',*,*,#13114,.F.);
#17989=ORIENTED_EDGE('',*,*,#13117,.F.);
#17990=ORIENTED_EDGE('',*,*,#13120,.F.);
#17991=ORIENTED_EDGE('',*,*,#13176,.F.);
#17992=ORIENTED_EDGE('',*,*,#13119,.T.);
#17993=ORIENTED_EDGE('',*,*,#13170,.T.);
#17994=ORIENTED_EDGE('',*,*,#13177,.F.);
#17995=ORIENTED_EDGE('',*,*,#13176,.T.);
#17996=ORIENTED_EDGE('',*,*,#13178,.T.);
#17997=ORIENTED_EDGE('',*,*,#13179,.F.);
#17998=ORIENTED_EDGE('',*,*,#13178,.F.);
#17999=ORIENTED_EDGE('',*,*,#13180,.F.);
#18000=ORIENTED_EDGE('',*,*,#13181,.F.);
#18001=ORIENTED_EDGE('',*,*,#13182,.T.);
#18002=ORIENTED_EDGE('',*,*,#13183,.T.);
#18003=ORIENTED_EDGE('',*,*,#13184,.F.);
#18004=ORIENTED_EDGE('',*,*,#13183,.F.);
#18005=ORIENTED_EDGE('',*,*,#13185,.F.);
#18006=ORIENTED_EDGE('',*,*,#13186,.F.);
#18007=ORIENTED_EDGE('',*,*,#13185,.T.);
#18008=ORIENTED_EDGE('',*,*,#13182,.F.);
#18009=ORIENTED_EDGE('',*,*,#13187,.F.);
#18010=ORIENTED_EDGE('',*,*,#13188,.F.);
#18011=ORIENTED_EDGE('',*,*,#13187,.T.);
#18012=ORIENTED_EDGE('',*,*,#13181,.T.);
#18013=ORIENTED_EDGE('',*,*,#13189,.F.);
#18014=ORIENTED_EDGE('',*,*,#13190,.F.);
#18015=ORIENTED_EDGE('',*,*,#13191,.T.);
#18016=ORIENTED_EDGE('',*,*,#13192,.T.);
#18017=ORIENTED_EDGE('',*,*,#13193,.F.);
#18018=ORIENTED_EDGE('',*,*,#13192,.F.);
#18019=ORIENTED_EDGE('',*,*,#13194,.F.);
#18020=ORIENTED_EDGE('',*,*,#13195,.F.);
#18021=ORIENTED_EDGE('',*,*,#13194,.T.);
#18022=ORIENTED_EDGE('',*,*,#13191,.F.);
#18023=ORIENTED_EDGE('',*,*,#13196,.F.);
#18024=ORIENTED_EDGE('',*,*,#13197,.F.);
#18025=ORIENTED_EDGE('',*,*,#13196,.T.);
#18026=ORIENTED_EDGE('',*,*,#13190,.T.);
#18027=ORIENTED_EDGE('',*,*,#13198,.F.);
#18028=ORIENTED_EDGE('',*,*,#13199,.F.);
#18029=ORIENTED_EDGE('',*,*,#13200,.T.);
#18030=ORIENTED_EDGE('',*,*,#13201,.T.);
#18031=ORIENTED_EDGE('',*,*,#13202,.F.);
#18032=ORIENTED_EDGE('',*,*,#13201,.F.);
#18033=ORIENTED_EDGE('',*,*,#13203,.F.);
#18034=ORIENTED_EDGE('',*,*,#13204,.F.);
#18035=ORIENTED_EDGE('',*,*,#13203,.T.);
#18036=ORIENTED_EDGE('',*,*,#13200,.F.);
#18037=ORIENTED_EDGE('',*,*,#13205,.F.);
#18038=ORIENTED_EDGE('',*,*,#13206,.F.);
#18039=ORIENTED_EDGE('',*,*,#13205,.T.);
#18040=ORIENTED_EDGE('',*,*,#13199,.T.);
#18041=ORIENTED_EDGE('',*,*,#13207,.F.);
#18042=ORIENTED_EDGE('',*,*,#13208,.F.);
#18043=ORIENTED_EDGE('',*,*,#13209,.T.);
#18044=ORIENTED_EDGE('',*,*,#13210,.T.);
#18045=ORIENTED_EDGE('',*,*,#13211,.F.);
#18046=ORIENTED_EDGE('',*,*,#13210,.F.);
#18047=ORIENTED_EDGE('',*,*,#13212,.F.);
#18048=ORIENTED_EDGE('',*,*,#13213,.F.);
#18049=ORIENTED_EDGE('',*,*,#13212,.T.);
#18050=ORIENTED_EDGE('',*,*,#13209,.F.);
#18051=ORIENTED_EDGE('',*,*,#13214,.F.);
#18052=ORIENTED_EDGE('',*,*,#13215,.F.);
#18053=ORIENTED_EDGE('',*,*,#13214,.T.);
#18054=ORIENTED_EDGE('',*,*,#13208,.T.);
#18055=ORIENTED_EDGE('',*,*,#13216,.F.);
#18056=ORIENTED_EDGE('',*,*,#13217,.F.);
#18057=ORIENTED_EDGE('',*,*,#13218,.T.);
#18058=ORIENTED_EDGE('',*,*,#13219,.T.);
#18059=ORIENTED_EDGE('',*,*,#13220,.F.);
#18060=ORIENTED_EDGE('',*,*,#13219,.F.);
#18061=ORIENTED_EDGE('',*,*,#13221,.F.);
#18062=ORIENTED_EDGE('',*,*,#13222,.F.);
#18063=ORIENTED_EDGE('',*,*,#13221,.T.);
#18064=ORIENTED_EDGE('',*,*,#13218,.F.);
#18065=ORIENTED_EDGE('',*,*,#13223,.F.);
#18066=ORIENTED_EDGE('',*,*,#13224,.F.);
#18067=ORIENTED_EDGE('',*,*,#13223,.T.);
#18068=ORIENTED_EDGE('',*,*,#13217,.T.);
#18069=ORIENTED_EDGE('',*,*,#13225,.F.);
#18070=ORIENTED_EDGE('',*,*,#13226,.F.);
#18071=ORIENTED_EDGE('',*,*,#13227,.T.);
#18072=ORIENTED_EDGE('',*,*,#13228,.T.);
#18073=ORIENTED_EDGE('',*,*,#13229,.F.);
#18074=ORIENTED_EDGE('',*,*,#13228,.F.);
#18075=ORIENTED_EDGE('',*,*,#13230,.F.);
#18076=ORIENTED_EDGE('',*,*,#13231,.F.);
#18077=ORIENTED_EDGE('',*,*,#13230,.T.);
#18078=ORIENTED_EDGE('',*,*,#13227,.F.);
#18079=ORIENTED_EDGE('',*,*,#13232,.F.);
#18080=ORIENTED_EDGE('',*,*,#13233,.F.);
#18081=ORIENTED_EDGE('',*,*,#13232,.T.);
#18082=ORIENTED_EDGE('',*,*,#13226,.T.);
#18083=ORIENTED_EDGE('',*,*,#13234,.F.);
#18084=ORIENTED_EDGE('',*,*,#13235,.F.);
#18085=ORIENTED_EDGE('',*,*,#13236,.T.);
#18086=ORIENTED_EDGE('',*,*,#13237,.T.);
#18087=ORIENTED_EDGE('',*,*,#13238,.F.);
#18088=ORIENTED_EDGE('',*,*,#13237,.F.);
#18089=ORIENTED_EDGE('',*,*,#13239,.F.);
#18090=ORIENTED_EDGE('',*,*,#13240,.F.);
#18091=ORIENTED_EDGE('',*,*,#13239,.T.);
#18092=ORIENTED_EDGE('',*,*,#13236,.F.);
#18093=ORIENTED_EDGE('',*,*,#13241,.F.);
#18094=ORIENTED_EDGE('',*,*,#13242,.F.);
#18095=ORIENTED_EDGE('',*,*,#13241,.T.);
#18096=ORIENTED_EDGE('',*,*,#13235,.T.);
#18097=ORIENTED_EDGE('',*,*,#13243,.F.);
#18098=ORIENTED_EDGE('',*,*,#13244,.F.);
#18099=ORIENTED_EDGE('',*,*,#13245,.T.);
#18100=ORIENTED_EDGE('',*,*,#13246,.T.);
#18101=ORIENTED_EDGE('',*,*,#13247,.F.);
#18102=ORIENTED_EDGE('',*,*,#13246,.F.);
#18103=ORIENTED_EDGE('',*,*,#13248,.F.);
#18104=ORIENTED_EDGE('',*,*,#13249,.F.);
#18105=ORIENTED_EDGE('',*,*,#13248,.T.);
#18106=ORIENTED_EDGE('',*,*,#13245,.F.);
#18107=ORIENTED_EDGE('',*,*,#13250,.F.);
#18108=ORIENTED_EDGE('',*,*,#13251,.F.);
#18109=ORIENTED_EDGE('',*,*,#13250,.T.);
#18110=ORIENTED_EDGE('',*,*,#13244,.T.);
#18111=ORIENTED_EDGE('',*,*,#13252,.F.);
#18112=ORIENTED_EDGE('',*,*,#13253,.F.);
#18113=ORIENTED_EDGE('',*,*,#13254,.T.);
#18114=ORIENTED_EDGE('',*,*,#13255,.T.);
#18115=ORIENTED_EDGE('',*,*,#13256,.F.);
#18116=ORIENTED_EDGE('',*,*,#13255,.F.);
#18117=ORIENTED_EDGE('',*,*,#13257,.F.);
#18118=ORIENTED_EDGE('',*,*,#13258,.F.);
#18119=ORIENTED_EDGE('',*,*,#13257,.T.);
#18120=ORIENTED_EDGE('',*,*,#13254,.F.);
#18121=ORIENTED_EDGE('',*,*,#13259,.F.);
#18122=ORIENTED_EDGE('',*,*,#13260,.F.);
#18123=ORIENTED_EDGE('',*,*,#13259,.T.);
#18124=ORIENTED_EDGE('',*,*,#13253,.T.);
#18125=ORIENTED_EDGE('',*,*,#13261,.F.);
#18126=ORIENTED_EDGE('',*,*,#13262,.F.);
#18127=ORIENTED_EDGE('',*,*,#13263,.T.);
#18128=ORIENTED_EDGE('',*,*,#13264,.T.);
#18129=ORIENTED_EDGE('',*,*,#13265,.F.);
#18130=ORIENTED_EDGE('',*,*,#13264,.F.);
#18131=ORIENTED_EDGE('',*,*,#13266,.F.);
#18132=ORIENTED_EDGE('',*,*,#13267,.F.);
#18133=ORIENTED_EDGE('',*,*,#13266,.T.);
#18134=ORIENTED_EDGE('',*,*,#13263,.F.);
#18135=ORIENTED_EDGE('',*,*,#13268,.F.);
#18136=ORIENTED_EDGE('',*,*,#13269,.F.);
#18137=ORIENTED_EDGE('',*,*,#13268,.T.);
#18138=ORIENTED_EDGE('',*,*,#13262,.T.);
#18139=ORIENTED_EDGE('',*,*,#13270,.F.);
#18140=ORIENTED_EDGE('',*,*,#13271,.F.);
#18141=ORIENTED_EDGE('',*,*,#13272,.T.);
#18142=ORIENTED_EDGE('',*,*,#13273,.T.);
#18143=ORIENTED_EDGE('',*,*,#13274,.F.);
#18144=ORIENTED_EDGE('',*,*,#13273,.F.);
#18145=ORIENTED_EDGE('',*,*,#13275,.F.);
#18146=ORIENTED_EDGE('',*,*,#13276,.F.);
#18147=ORIENTED_EDGE('',*,*,#13275,.T.);
#18148=ORIENTED_EDGE('',*,*,#13272,.F.);
#18149=ORIENTED_EDGE('',*,*,#13277,.F.);
#18150=ORIENTED_EDGE('',*,*,#13278,.F.);
#18151=ORIENTED_EDGE('',*,*,#13277,.T.);
#18152=ORIENTED_EDGE('',*,*,#13271,.T.);
#18153=ORIENTED_EDGE('',*,*,#13279,.F.);
#18154=ORIENTED_EDGE('',*,*,#13280,.F.);
#18155=ORIENTED_EDGE('',*,*,#13281,.T.);
#18156=ORIENTED_EDGE('',*,*,#13282,.T.);
#18157=ORIENTED_EDGE('',*,*,#13283,.F.);
#18158=ORIENTED_EDGE('',*,*,#13282,.F.);
#18159=ORIENTED_EDGE('',*,*,#13284,.F.);
#18160=ORIENTED_EDGE('',*,*,#13285,.F.);
#18161=ORIENTED_EDGE('',*,*,#13286,.F.);
#18162=ORIENTED_EDGE('',*,*,#13284,.T.);
#18163=ORIENTED_EDGE('',*,*,#13281,.F.);
#18164=ORIENTED_EDGE('',*,*,#13287,.F.);
#18165=ORIENTED_EDGE('',*,*,#13288,.F.);
#18166=ORIENTED_EDGE('',*,*,#13287,.T.);
#18167=ORIENTED_EDGE('',*,*,#13280,.T.);
#18168=ORIENTED_EDGE('',*,*,#13289,.F.);
#18169=ORIENTED_EDGE('',*,*,#13290,.F.);
#18170=ORIENTED_EDGE('',*,*,#13291,.F.);
#18171=ORIENTED_EDGE('',*,*,#13292,.T.);
#18172=ORIENTED_EDGE('',*,*,#13293,.T.);
#18173=ORIENTED_EDGE('',*,*,#13294,.F.);
#18174=ORIENTED_EDGE('',*,*,#13293,.F.);
#18175=ORIENTED_EDGE('',*,*,#13295,.F.);
#18176=ORIENTED_EDGE('',*,*,#13296,.F.);
#18177=ORIENTED_EDGE('',*,*,#13295,.T.);
#18178=ORIENTED_EDGE('',*,*,#13292,.F.);
#18179=ORIENTED_EDGE('',*,*,#13297,.F.);
#18180=ORIENTED_EDGE('',*,*,#13298,.F.);
#18181=ORIENTED_EDGE('',*,*,#13297,.T.);
#18182=ORIENTED_EDGE('',*,*,#13291,.T.);
#18183=ORIENTED_EDGE('',*,*,#13299,.F.);
#18184=ORIENTED_EDGE('',*,*,#13300,.F.);
#18185=ORIENTED_EDGE('',*,*,#13301,.T.);
#18186=ORIENTED_EDGE('',*,*,#13302,.T.);
#18187=ORIENTED_EDGE('',*,*,#13303,.F.);
#18188=ORIENTED_EDGE('',*,*,#13302,.F.);
#18189=ORIENTED_EDGE('',*,*,#13304,.F.);
#18190=ORIENTED_EDGE('',*,*,#13305,.F.);
#18191=ORIENTED_EDGE('',*,*,#13304,.T.);
#18192=ORIENTED_EDGE('',*,*,#13301,.F.);
#18193=ORIENTED_EDGE('',*,*,#13306,.F.);
#18194=ORIENTED_EDGE('',*,*,#13307,.F.);
#18195=ORIENTED_EDGE('',*,*,#13306,.T.);
#18196=ORIENTED_EDGE('',*,*,#13300,.T.);
#18197=ORIENTED_EDGE('',*,*,#13308,.F.);
#18198=ORIENTED_EDGE('',*,*,#13309,.F.);
#18199=ORIENTED_EDGE('',*,*,#13310,.T.);
#18200=ORIENTED_EDGE('',*,*,#13311,.T.);
#18201=ORIENTED_EDGE('',*,*,#13312,.F.);
#18202=ORIENTED_EDGE('',*,*,#13311,.F.);
#18203=ORIENTED_EDGE('',*,*,#13313,.F.);
#18204=ORIENTED_EDGE('',*,*,#13314,.F.);
#18205=ORIENTED_EDGE('',*,*,#13313,.T.);
#18206=ORIENTED_EDGE('',*,*,#13310,.F.);
#18207=ORIENTED_EDGE('',*,*,#13315,.F.);
#18208=ORIENTED_EDGE('',*,*,#13316,.F.);
#18209=ORIENTED_EDGE('',*,*,#13315,.T.);
#18210=ORIENTED_EDGE('',*,*,#13309,.T.);
#18211=ORIENTED_EDGE('',*,*,#13317,.F.);
#18212=ORIENTED_EDGE('',*,*,#13318,.F.);
#18213=ORIENTED_EDGE('',*,*,#13319,.T.);
#18214=ORIENTED_EDGE('',*,*,#13320,.T.);
#18215=ORIENTED_EDGE('',*,*,#13321,.F.);
#18216=ORIENTED_EDGE('',*,*,#13320,.F.);
#18217=ORIENTED_EDGE('',*,*,#13322,.F.);
#18218=ORIENTED_EDGE('',*,*,#13323,.F.);
#18219=ORIENTED_EDGE('',*,*,#13322,.T.);
#18220=ORIENTED_EDGE('',*,*,#13319,.F.);
#18221=ORIENTED_EDGE('',*,*,#13324,.F.);
#18222=ORIENTED_EDGE('',*,*,#13325,.F.);
#18223=ORIENTED_EDGE('',*,*,#13324,.T.);
#18224=ORIENTED_EDGE('',*,*,#13318,.T.);
#18225=ORIENTED_EDGE('',*,*,#13326,.F.);
#18226=ORIENTED_EDGE('',*,*,#13327,.F.);
#18227=ORIENTED_EDGE('',*,*,#13328,.T.);
#18228=ORIENTED_EDGE('',*,*,#13329,.T.);
#18229=ORIENTED_EDGE('',*,*,#13330,.F.);
#18230=ORIENTED_EDGE('',*,*,#13329,.F.);
#18231=ORIENTED_EDGE('',*,*,#13331,.F.);
#18232=ORIENTED_EDGE('',*,*,#13332,.F.);
#18233=ORIENTED_EDGE('',*,*,#13331,.T.);
#18234=ORIENTED_EDGE('',*,*,#13328,.F.);
#18235=ORIENTED_EDGE('',*,*,#13333,.F.);
#18236=ORIENTED_EDGE('',*,*,#13334,.F.);
#18237=ORIENTED_EDGE('',*,*,#13333,.T.);
#18238=ORIENTED_EDGE('',*,*,#13327,.T.);
#18239=ORIENTED_EDGE('',*,*,#13335,.F.);
#18240=ORIENTED_EDGE('',*,*,#13336,.F.);
#18241=ORIENTED_EDGE('',*,*,#13337,.T.);
#18242=ORIENTED_EDGE('',*,*,#13338,.T.);
#18243=ORIENTED_EDGE('',*,*,#13339,.F.);
#18244=ORIENTED_EDGE('',*,*,#13338,.F.);
#18245=ORIENTED_EDGE('',*,*,#13340,.F.);
#18246=ORIENTED_EDGE('',*,*,#13341,.F.);
#18247=ORIENTED_EDGE('',*,*,#13340,.T.);
#18248=ORIENTED_EDGE('',*,*,#13337,.F.);
#18249=ORIENTED_EDGE('',*,*,#13342,.F.);
#18250=ORIENTED_EDGE('',*,*,#13343,.F.);
#18251=ORIENTED_EDGE('',*,*,#13342,.T.);
#18252=ORIENTED_EDGE('',*,*,#13336,.T.);
#18253=ORIENTED_EDGE('',*,*,#13344,.F.);
#18254=ORIENTED_EDGE('',*,*,#13345,.F.);
#18255=ORIENTED_EDGE('',*,*,#13346,.T.);
#18256=ORIENTED_EDGE('',*,*,#13347,.T.);
#18257=ORIENTED_EDGE('',*,*,#13348,.F.);
#18258=ORIENTED_EDGE('',*,*,#13347,.F.);
#18259=ORIENTED_EDGE('',*,*,#13349,.F.);
#18260=ORIENTED_EDGE('',*,*,#13350,.F.);
#18261=ORIENTED_EDGE('',*,*,#13349,.T.);
#18262=ORIENTED_EDGE('',*,*,#13346,.F.);
#18263=ORIENTED_EDGE('',*,*,#13351,.F.);
#18264=ORIENTED_EDGE('',*,*,#13352,.F.);
#18265=ORIENTED_EDGE('',*,*,#13351,.T.);
#18266=ORIENTED_EDGE('',*,*,#13345,.T.);
#18267=ORIENTED_EDGE('',*,*,#13353,.F.);
#18268=ORIENTED_EDGE('',*,*,#13354,.F.);
#18269=ORIENTED_EDGE('',*,*,#13355,.T.);
#18270=ORIENTED_EDGE('',*,*,#13356,.T.);
#18271=ORIENTED_EDGE('',*,*,#13357,.F.);
#18272=ORIENTED_EDGE('',*,*,#13356,.F.);
#18273=ORIENTED_EDGE('',*,*,#13358,.F.);
#18274=ORIENTED_EDGE('',*,*,#13359,.F.);
#18275=ORIENTED_EDGE('',*,*,#13358,.T.);
#18276=ORIENTED_EDGE('',*,*,#13355,.F.);
#18277=ORIENTED_EDGE('',*,*,#13360,.F.);
#18278=ORIENTED_EDGE('',*,*,#13361,.F.);
#18279=ORIENTED_EDGE('',*,*,#13360,.T.);
#18280=ORIENTED_EDGE('',*,*,#13354,.T.);
#18281=ORIENTED_EDGE('',*,*,#13362,.F.);
#18282=ORIENTED_EDGE('',*,*,#13363,.F.);
#18283=ORIENTED_EDGE('',*,*,#13364,.T.);
#18284=ORIENTED_EDGE('',*,*,#13365,.T.);
#18285=ORIENTED_EDGE('',*,*,#13366,.F.);
#18286=ORIENTED_EDGE('',*,*,#13365,.F.);
#18287=ORIENTED_EDGE('',*,*,#13367,.F.);
#18288=ORIENTED_EDGE('',*,*,#13368,.F.);
#18289=ORIENTED_EDGE('',*,*,#13367,.T.);
#18290=ORIENTED_EDGE('',*,*,#13364,.F.);
#18291=ORIENTED_EDGE('',*,*,#13369,.F.);
#18292=ORIENTED_EDGE('',*,*,#13370,.F.);
#18293=ORIENTED_EDGE('',*,*,#13369,.T.);
#18294=ORIENTED_EDGE('',*,*,#13363,.T.);
#18295=ORIENTED_EDGE('',*,*,#13371,.F.);
#18296=ORIENTED_EDGE('',*,*,#13372,.F.);
#18297=ORIENTED_EDGE('',*,*,#13373,.T.);
#18298=ORIENTED_EDGE('',*,*,#13374,.T.);
#18299=ORIENTED_EDGE('',*,*,#13375,.F.);
#18300=ORIENTED_EDGE('',*,*,#13374,.F.);
#18301=ORIENTED_EDGE('',*,*,#13376,.F.);
#18302=ORIENTED_EDGE('',*,*,#13377,.F.);
#18303=ORIENTED_EDGE('',*,*,#13376,.T.);
#18304=ORIENTED_EDGE('',*,*,#13373,.F.);
#18305=ORIENTED_EDGE('',*,*,#13378,.F.);
#18306=ORIENTED_EDGE('',*,*,#13379,.F.);
#18307=ORIENTED_EDGE('',*,*,#13378,.T.);
#18308=ORIENTED_EDGE('',*,*,#13372,.T.);
#18309=ORIENTED_EDGE('',*,*,#13380,.F.);
#18310=ORIENTED_EDGE('',*,*,#13381,.F.);
#18311=ORIENTED_EDGE('',*,*,#13382,.T.);
#18312=ORIENTED_EDGE('',*,*,#13383,.T.);
#18313=ORIENTED_EDGE('',*,*,#13384,.F.);
#18314=ORIENTED_EDGE('',*,*,#13383,.F.);
#18315=ORIENTED_EDGE('',*,*,#13385,.F.);
#18316=ORIENTED_EDGE('',*,*,#13386,.F.);
#18317=ORIENTED_EDGE('',*,*,#13385,.T.);
#18318=ORIENTED_EDGE('',*,*,#13382,.F.);
#18319=ORIENTED_EDGE('',*,*,#13387,.F.);
#18320=ORIENTED_EDGE('',*,*,#13388,.F.);
#18321=ORIENTED_EDGE('',*,*,#13387,.T.);
#18322=ORIENTED_EDGE('',*,*,#13381,.T.);
#18323=ORIENTED_EDGE('',*,*,#13389,.F.);
#18324=ORIENTED_EDGE('',*,*,#13390,.F.);
#18325=ORIENTED_EDGE('',*,*,#13391,.T.);
#18326=ORIENTED_EDGE('',*,*,#13392,.T.);
#18327=ORIENTED_EDGE('',*,*,#13393,.F.);
#18328=ORIENTED_EDGE('',*,*,#13392,.F.);
#18329=ORIENTED_EDGE('',*,*,#13394,.F.);
#18330=ORIENTED_EDGE('',*,*,#13395,.F.);
#18331=ORIENTED_EDGE('',*,*,#13394,.T.);
#18332=ORIENTED_EDGE('',*,*,#13391,.F.);
#18333=ORIENTED_EDGE('',*,*,#13396,.F.);
#18334=ORIENTED_EDGE('',*,*,#13397,.F.);
#18335=ORIENTED_EDGE('',*,*,#13396,.T.);
#18336=ORIENTED_EDGE('',*,*,#13390,.T.);
#18337=ORIENTED_EDGE('',*,*,#13398,.F.);
#18338=ORIENTED_EDGE('',*,*,#13080,.F.);
#18339=ORIENTED_EDGE('',*,*,#13399,.T.);
#18340=ORIENTED_EDGE('',*,*,#13398,.T.);
#18341=ORIENTED_EDGE('',*,*,#13399,.F.);
#18342=ORIENTED_EDGE('',*,*,#13400,.F.);
#18343=ORIENTED_EDGE('',*,*,#13177,.T.);
#18344=ORIENTED_EDGE('',*,*,#13169,.T.);
#18345=ORIENTED_EDGE('',*,*,#13124,.T.);
#18346=ORIENTED_EDGE('',*,*,#13175,.T.);
#18347=ORIENTED_EDGE('',*,*,#13401,.F.);
#18348=ORIENTED_EDGE('',*,*,#13402,.T.);
#18349=ORIENTED_EDGE('',*,*,#13400,.T.);
#18350=ORIENTED_EDGE('',*,*,#13402,.F.);
#18351=ORIENTED_EDGE('',*,*,#13403,.F.);
#18352=ORIENTED_EDGE('',*,*,#13404,.T.);
#18353=ORIENTED_EDGE('',*,*,#13285,.T.);
#18354=ORIENTED_EDGE('',*,*,#13286,.T.);
#18355=ORIENTED_EDGE('',*,*,#13288,.T.);
#18356=ORIENTED_EDGE('',*,*,#13405,.T.);
#18357=ORIENTED_EDGE('',*,*,#13401,.T.);
#18358=ORIENTED_EDGE('',*,*,#13405,.F.);
#18359=ORIENTED_EDGE('',*,*,#13289,.T.);
#18360=ORIENTED_EDGE('',*,*,#13279,.T.);
#18361=ORIENTED_EDGE('',*,*,#13283,.T.);
#18362=ORIENTED_EDGE('',*,*,#13404,.F.);
#18363=ORIENTED_EDGE('',*,*,#13186,.T.);
#18364=ORIENTED_EDGE('',*,*,#13188,.T.);
#18365=ORIENTED_EDGE('',*,*,#13180,.T.);
#18366=ORIENTED_EDGE('',*,*,#13184,.T.);
#18367=ORIENTED_EDGE('',*,*,#13195,.T.);
#18368=ORIENTED_EDGE('',*,*,#13197,.T.);
#18369=ORIENTED_EDGE('',*,*,#13189,.T.);
#18370=ORIENTED_EDGE('',*,*,#13193,.T.);
#18371=ORIENTED_EDGE('',*,*,#13204,.T.);
#18372=ORIENTED_EDGE('',*,*,#13206,.T.);
#18373=ORIENTED_EDGE('',*,*,#13198,.T.);
#18374=ORIENTED_EDGE('',*,*,#13202,.T.);
#18375=ORIENTED_EDGE('',*,*,#13213,.T.);
#18376=ORIENTED_EDGE('',*,*,#13215,.T.);
#18377=ORIENTED_EDGE('',*,*,#13207,.T.);
#18378=ORIENTED_EDGE('',*,*,#13211,.T.);
#18379=ORIENTED_EDGE('',*,*,#13222,.T.);
#18380=ORIENTED_EDGE('',*,*,#13224,.T.);
#18381=ORIENTED_EDGE('',*,*,#13216,.T.);
#18382=ORIENTED_EDGE('',*,*,#13220,.T.);
#18383=ORIENTED_EDGE('',*,*,#13231,.T.);
#18384=ORIENTED_EDGE('',*,*,#13233,.T.);
#18385=ORIENTED_EDGE('',*,*,#13225,.T.);
#18386=ORIENTED_EDGE('',*,*,#13229,.T.);
#18387=ORIENTED_EDGE('',*,*,#13240,.T.);
#18388=ORIENTED_EDGE('',*,*,#13242,.T.);
#18389=ORIENTED_EDGE('',*,*,#13234,.T.);
#18390=ORIENTED_EDGE('',*,*,#13238,.T.);
#18391=ORIENTED_EDGE('',*,*,#13249,.T.);
#18392=ORIENTED_EDGE('',*,*,#13251,.T.);
#18393=ORIENTED_EDGE('',*,*,#13243,.T.);
#18394=ORIENTED_EDGE('',*,*,#13247,.T.);
#18395=ORIENTED_EDGE('',*,*,#13258,.T.);
#18396=ORIENTED_EDGE('',*,*,#13260,.T.);
#18397=ORIENTED_EDGE('',*,*,#13252,.T.);
#18398=ORIENTED_EDGE('',*,*,#13256,.T.);
#18399=ORIENTED_EDGE('',*,*,#13267,.T.);
#18400=ORIENTED_EDGE('',*,*,#13269,.T.);
#18401=ORIENTED_EDGE('',*,*,#13261,.T.);
#18402=ORIENTED_EDGE('',*,*,#13265,.T.);
#18403=ORIENTED_EDGE('',*,*,#13276,.T.);
#18404=ORIENTED_EDGE('',*,*,#13278,.T.);
#18405=ORIENTED_EDGE('',*,*,#13270,.T.);
#18406=ORIENTED_EDGE('',*,*,#13274,.T.);
#18407=ORIENTED_EDGE('',*,*,#13296,.T.);
#18408=ORIENTED_EDGE('',*,*,#13298,.T.);
#18409=ORIENTED_EDGE('',*,*,#13290,.T.);
#18410=ORIENTED_EDGE('',*,*,#13294,.T.);
#18411=ORIENTED_EDGE('',*,*,#13305,.T.);
#18412=ORIENTED_EDGE('',*,*,#13307,.T.);
#18413=ORIENTED_EDGE('',*,*,#13299,.T.);
#18414=ORIENTED_EDGE('',*,*,#13303,.T.);
#18415=ORIENTED_EDGE('',*,*,#13314,.T.);
#18416=ORIENTED_EDGE('',*,*,#13316,.T.);
#18417=ORIENTED_EDGE('',*,*,#13308,.T.);
#18418=ORIENTED_EDGE('',*,*,#13312,.T.);
#18419=ORIENTED_EDGE('',*,*,#13323,.T.);
#18420=ORIENTED_EDGE('',*,*,#13325,.T.);
#18421=ORIENTED_EDGE('',*,*,#13317,.T.);
#18422=ORIENTED_EDGE('',*,*,#13321,.T.);
#18423=ORIENTED_EDGE('',*,*,#13332,.T.);
#18424=ORIENTED_EDGE('',*,*,#13334,.T.);
#18425=ORIENTED_EDGE('',*,*,#13326,.T.);
#18426=ORIENTED_EDGE('',*,*,#13330,.T.);
#18427=ORIENTED_EDGE('',*,*,#13341,.T.);
#18428=ORIENTED_EDGE('',*,*,#13343,.T.);
#18429=ORIENTED_EDGE('',*,*,#13335,.T.);
#18430=ORIENTED_EDGE('',*,*,#13339,.T.);
#18431=ORIENTED_EDGE('',*,*,#13350,.T.);
#18432=ORIENTED_EDGE('',*,*,#13352,.T.);
#18433=ORIENTED_EDGE('',*,*,#13344,.T.);
#18434=ORIENTED_EDGE('',*,*,#13348,.T.);
#18435=ORIENTED_EDGE('',*,*,#13359,.T.);
#18436=ORIENTED_EDGE('',*,*,#13361,.T.);
#18437=ORIENTED_EDGE('',*,*,#13353,.T.);
#18438=ORIENTED_EDGE('',*,*,#13357,.T.);
#18439=ORIENTED_EDGE('',*,*,#13368,.T.);
#18440=ORIENTED_EDGE('',*,*,#13370,.T.);
#18441=ORIENTED_EDGE('',*,*,#13362,.T.);
#18442=ORIENTED_EDGE('',*,*,#13366,.T.);
#18443=ORIENTED_EDGE('',*,*,#13377,.T.);
#18444=ORIENTED_EDGE('',*,*,#13379,.T.);
#18445=ORIENTED_EDGE('',*,*,#13371,.T.);
#18446=ORIENTED_EDGE('',*,*,#13375,.T.);
#18447=ORIENTED_EDGE('',*,*,#13386,.T.);
#18448=ORIENTED_EDGE('',*,*,#13388,.T.);
#18449=ORIENTED_EDGE('',*,*,#13380,.T.);
#18450=ORIENTED_EDGE('',*,*,#13384,.T.);
#18451=ORIENTED_EDGE('',*,*,#13395,.T.);
#18452=ORIENTED_EDGE('',*,*,#13397,.T.);
#18453=ORIENTED_EDGE('',*,*,#13389,.T.);
#18454=ORIENTED_EDGE('',*,*,#13393,.T.);
#18455=ORIENTED_EDGE('',*,*,#13406,.F.);
#18456=ORIENTED_EDGE('',*,*,#13407,.T.);
#18457=ORIENTED_EDGE('',*,*,#13403,.T.);
#18458=ORIENTED_EDGE('',*,*,#13407,.F.);
#18459=ORIENTED_EDGE('',*,*,#13406,.T.);
#18460=ORIENTED_EDGE('',*,*,#13179,.T.);
#21959=CONICAL_SURFACE('',#24635,0.1,1.27933953231703);
#21960=CONICAL_SURFACE('',#24785,0.18,0.785398163397448);
#21961=CONICAL_SURFACE('',#24788,0.575,0.785398163397448);
#21962=CONICAL_SURFACE('',#24792,0.55,0.785398163397448);
#22595=ADVANCED_FACE('',(#2856),#1053,.T.);
#22596=ADVANCED_FACE('',(#2857),#1054,.T.);
#22597=ADVANCED_FACE('',(#2858),#1055,.T.);
#22598=ADVANCED_FACE('',(#2859),#1056,.T.);
#22599=ADVANCED_FACE('',(#2860),#1057,.T.);
#22600=ADVANCED_FACE('',(#2861),#1058,.T.);
#22601=ADVANCED_FACE('',(#2862),#1059,.T.);
#22602=ADVANCED_FACE('',(#2863),#1060,.T.);
#22603=ADVANCED_FACE('',(#2864),#1061,.T.);
#22604=ADVANCED_FACE('',(#2865),#1062,.T.);
#22605=ADVANCED_FACE('',(#2866),#1063,.T.);
#22606=ADVANCED_FACE('',(#2867),#1064,.T.);
#22607=ADVANCED_FACE('',(#2868),#1065,.T.);
#22608=ADVANCED_FACE('',(#2869),#1066,.T.);
#22609=ADVANCED_FACE('',(#2870),#1067,.T.);
#22610=ADVANCED_FACE('',(#2871),#1068,.T.);
#22611=ADVANCED_FACE('',(#2872),#1069,.T.);
#22612=ADVANCED_FACE('',(#2873),#1070,.T.);
#22613=ADVANCED_FACE('',(#2874),#1071,.T.);
#22614=ADVANCED_FACE('',(#2875),#1072,.T.);
#22615=ADVANCED_FACE('',(#2876),#1073,.T.);
#22616=ADVANCED_FACE('',(#2877),#1074,.T.);
#22617=ADVANCED_FACE('',(#2878),#1075,.T.);
#22618=ADVANCED_FACE('',(#2879),#1076,.T.);
#22619=ADVANCED_FACE('',(#2880),#1077,.T.);
#22620=ADVANCED_FACE('',(#2881),#1078,.T.);
#22621=ADVANCED_FACE('',(#2882),#1079,.T.);
#22622=ADVANCED_FACE('',(#2883),#1080,.T.);
#22623=ADVANCED_FACE('',(#2884),#1081,.T.);
#22624=ADVANCED_FACE('',(#2885),#365,.F.);
#22625=ADVANCED_FACE('',(#2886),#1776,.T.);
#22626=ADVANCED_FACE('',(#2887),#1082,.T.);
#22627=ADVANCED_FACE('',(#2888),#366,.F.);
#22628=ADVANCED_FACE('',(#2889),#1083,.T.);
#22629=ADVANCED_FACE('',(#2890),#21959,.F.);
#22630=ADVANCED_FACE('',(#2891),#1777,.F.);
#22631=ADVANCED_FACE('',(#2892),#1778,.F.);
#22632=ADVANCED_FACE('',(#2893),#1779,.F.);
#22633=ADVANCED_FACE('',(#2894),#1780,.T.);
#22634=ADVANCED_FACE('',(#2895),#1781,.F.);
#22635=ADVANCED_FACE('',(#2896),#1782,.F.);
#22636=ADVANCED_FACE('',(#2897),#1783,.F.);
#22637=ADVANCED_FACE('',(#2898),#1784,.T.);
#22638=ADVANCED_FACE('',(#2899),#1785,.F.);
#22639=ADVANCED_FACE('',(#2900),#1786,.F.);
#22640=ADVANCED_FACE('',(#2901),#1787,.F.);
#22641=ADVANCED_FACE('',(#2902),#1788,.T.);
#22642=ADVANCED_FACE('',(#2903),#1789,.F.);
#22643=ADVANCED_FACE('',(#2904),#1790,.F.);
#22644=ADVANCED_FACE('',(#2905),#1791,.F.);
#22645=ADVANCED_FACE('',(#2906),#1792,.T.);
#22646=ADVANCED_FACE('',(#2907),#1793,.F.);
#22647=ADVANCED_FACE('',(#2908),#1794,.F.);
#22648=ADVANCED_FACE('',(#2909),#1795,.F.);
#22649=ADVANCED_FACE('',(#2910),#1796,.T.);
#22650=ADVANCED_FACE('',(#2911),#1797,.F.);
#22651=ADVANCED_FACE('',(#2912),#1798,.F.);
#22652=ADVANCED_FACE('',(#2913),#1799,.F.);
#22653=ADVANCED_FACE('',(#2914),#1800,.T.);
#22654=ADVANCED_FACE('',(#2915),#1801,.F.);
#22655=ADVANCED_FACE('',(#2916),#1802,.F.);
#22656=ADVANCED_FACE('',(#2917),#1803,.F.);
#22657=ADVANCED_FACE('',(#2918),#1804,.T.);
#22658=ADVANCED_FACE('',(#2919),#1805,.F.);
#22659=ADVANCED_FACE('',(#2920),#1806,.F.);
#22660=ADVANCED_FACE('',(#2921),#1807,.F.);
#22661=ADVANCED_FACE('',(#2922),#1808,.T.);
#22662=ADVANCED_FACE('',(#2923),#1809,.F.);
#22663=ADVANCED_FACE('',(#2924),#1810,.F.);
#22664=ADVANCED_FACE('',(#2925),#1811,.F.);
#22665=ADVANCED_FACE('',(#2926),#1812,.T.);
#22666=ADVANCED_FACE('',(#2927),#1813,.F.);
#22667=ADVANCED_FACE('',(#2928),#1814,.F.);
#22668=ADVANCED_FACE('',(#2929),#1815,.F.);
#22669=ADVANCED_FACE('',(#2930),#1816,.T.);
#22670=ADVANCED_FACE('',(#2931),#1817,.F.);
#22671=ADVANCED_FACE('',(#2932),#1818,.F.);
#22672=ADVANCED_FACE('',(#2933),#1819,.F.);
#22673=ADVANCED_FACE('',(#2934),#1820,.T.);
#22674=ADVANCED_FACE('',(#2935),#1821,.F.);
#22675=ADVANCED_FACE('',(#2936),#1822,.F.);
#22676=ADVANCED_FACE('',(#2937),#1823,.F.);
#22677=ADVANCED_FACE('',(#2938),#1824,.T.);
#22678=ADVANCED_FACE('',(#2939),#1825,.F.);
#22679=ADVANCED_FACE('',(#2940),#1826,.F.);
#22680=ADVANCED_FACE('',(#2941),#1827,.F.);
#22681=ADVANCED_FACE('',(#2942),#1828,.T.);
#22682=ADVANCED_FACE('',(#2943),#1829,.F.);
#22683=ADVANCED_FACE('',(#2944),#1830,.F.);
#22684=ADVANCED_FACE('',(#2945),#1831,.F.);
#22685=ADVANCED_FACE('',(#2946),#1832,.T.);
#22686=ADVANCED_FACE('',(#2947),#1833,.F.);
#22687=ADVANCED_FACE('',(#2948),#1834,.F.);
#22688=ADVANCED_FACE('',(#2949),#1835,.F.);
#22689=ADVANCED_FACE('',(#2950),#1836,.T.);
#22690=ADVANCED_FACE('',(#2951),#1837,.F.);
#22691=ADVANCED_FACE('',(#2952),#1838,.F.);
#22692=ADVANCED_FACE('',(#2953),#1839,.F.);
#22693=ADVANCED_FACE('',(#2954),#1840,.T.);
#22694=ADVANCED_FACE('',(#2955),#1841,.F.);
#22695=ADVANCED_FACE('',(#2956),#1842,.F.);
#22696=ADVANCED_FACE('',(#2957),#1843,.F.);
#22697=ADVANCED_FACE('',(#2958),#1844,.T.);
#22698=ADVANCED_FACE('',(#2959),#1845,.F.);
#22699=ADVANCED_FACE('',(#2960),#1846,.F.);
#22700=ADVANCED_FACE('',(#2961),#1847,.F.);
#22701=ADVANCED_FACE('',(#2962),#1848,.T.);
#22702=ADVANCED_FACE('',(#2963),#1849,.F.);
#22703=ADVANCED_FACE('',(#2964),#1850,.F.);
#22704=ADVANCED_FACE('',(#2965),#1851,.F.);
#22705=ADVANCED_FACE('',(#2966),#1852,.T.);
#22706=ADVANCED_FACE('',(#2967),#1853,.F.);
#22707=ADVANCED_FACE('',(#2968),#1854,.F.);
#22708=ADVANCED_FACE('',(#2969),#1855,.F.);
#22709=ADVANCED_FACE('',(#2970),#1856,.T.);
#22710=ADVANCED_FACE('',(#2971),#1857,.F.);
#22711=ADVANCED_FACE('',(#2972),#1858,.F.);
#22712=ADVANCED_FACE('',(#2973),#1859,.F.);
#22713=ADVANCED_FACE('',(#2974),#1860,.T.);
#22714=ADVANCED_FACE('',(#2975),#1861,.F.);
#22715=ADVANCED_FACE('',(#2976),#1862,.F.);
#22716=ADVANCED_FACE('',(#2977),#1863,.F.);
#22717=ADVANCED_FACE('',(#2978),#1864,.T.);
#22718=ADVANCED_FACE('',(#2979),#1865,.F.);
#22719=ADVANCED_FACE('',(#2980),#1866,.F.);
#22720=ADVANCED_FACE('',(#2981),#1867,.F.);
#22721=ADVANCED_FACE('',(#2982),#1868,.T.);
#22722=ADVANCED_FACE('',(#2983),#1869,.F.);
#22723=ADVANCED_FACE('',(#2984),#1870,.F.);
#22724=ADVANCED_FACE('',(#2985),#1871,.F.);
#22725=ADVANCED_FACE('',(#2986),#1872,.T.);
#22726=ADVANCED_FACE('',(#2987),#1873,.T.);
#22727=ADVANCED_FACE('',(#2988),#21960,.T.);
#22728=ADVANCED_FACE('',(#2989,#1414),#1874,.T.);
#22729=ADVANCED_FACE('',(#2990),#21961,.T.);
#22730=ADVANCED_FACE('',(#2991,#1415,#1416,#1417,#1418,#1419,#1420,#1421,
#1422,#1423,#1424,#1425,#1426,#1427,#1428,#1429,#1430,#1431,#1432,#1433,
#1434,#1435,#1436,#1437),#1084,.T.);
#22731=ADVANCED_FACE('',(#2992),#21962,.T.);
#22732=ADVANCED_FACE('',(#2993,#1438),#1875,.T.);
#23315=CLOSED_SHELL('',(#22595,#22596,#22597,#22598,#22599,#22600,#22601,
#22602,#22603,#22604,#22605,#22606,#22607,#22608,#22609,#22610,#22611,#22612,
#22613,#22614,#22615,#22616,#22617,#22618,#22619,#22620,#22621,#22622,#22623,
#22624,#22625,#22626,#22627,#22628,#22629,#22630,#22631,#22632,#22633,#22634,
#22635,#22636,#22637,#22638,#22639,#22640,#22641,#22642,#22643,#22644,#22645,
#22646,#22647,#22648,#22649,#22650,#22651,#22652,#22653,#22654,#22655,#22656,
#22657,#22658,#22659,#22660,#22661,#22662,#22663,#22664,#22665,#22666,#22667,
#22668,#22669,#22670,#22671,#22672,#22673,#22674,#22675,#22676,#22677,#22678,
#22679,#22680,#22681,#22682,#22683,#22684,#22685,#22686,#22687,#22688,#22689,
#22690,#22691,#22692,#22693,#22694,#22695,#22696,#22697,#22698,#22699,#22700,
#22701,#22702,#22703,#22704,#22705,#22706,#22707,#22708,#22709,#22710,#22711,
#22712,#22713,#22714,#22715,#22716,#22717,#22718,#22719,#22720,#22721,#22722,
#22723,#22724,#22725,#22726,#22727,#22728,#22729,#22730,#22731,#22732));
#24595=AXIS2_PLACEMENT_3D('',#36156,#28698,#28699);
#24596=AXIS2_PLACEMENT_3D('',#36157,#28700,#28701);
#24597=AXIS2_PLACEMENT_3D('',#36176,#28703,#28704);
#24598=AXIS2_PLACEMENT_3D('',#36179,#28706,#28707);
#24599=AXIS2_PLACEMENT_3D('',#36181,#28708,#28709);
#24600=AXIS2_PLACEMENT_3D('',#36192,#28710,#28711);
#24601=AXIS2_PLACEMENT_3D('',#36240,#28713,#28714);
#24602=AXIS2_PLACEMENT_3D('',#36294,#28716,#28717);
#24603=AXIS2_PLACEMENT_3D('',#36342,#28719,#28720);
#24604=AXIS2_PLACEMENT_3D('',#36390,#28722,#28723);
#24605=AXIS2_PLACEMENT_3D('',#36438,#28725,#28726);
#24606=AXIS2_PLACEMENT_3D('',#36492,#28728,#28729);
#24607=AXIS2_PLACEMENT_3D('',#36540,#28731,#28732);
#24608=AXIS2_PLACEMENT_3D('',#36588,#28734,#28735);
#24609=AXIS2_PLACEMENT_3D('',#36642,#28737,#28738);
#24610=AXIS2_PLACEMENT_3D('',#36690,#28740,#28741);
#24611=AXIS2_PLACEMENT_3D('',#36738,#28743,#28744);
#24612=AXIS2_PLACEMENT_3D('',#36792,#28746,#28747);
#24613=AXIS2_PLACEMENT_3D('',#36840,#28749,#28750);
#24614=AXIS2_PLACEMENT_3D('',#36852,#28752,#28753);
#24615=AXIS2_PLACEMENT_3D('',#36858,#28754,#28755);
#24616=AXIS2_PLACEMENT_3D('',#36882,#28757,#28758);
#24617=AXIS2_PLACEMENT_3D('',#36907,#28760,#28761);
#24618=AXIS2_PLACEMENT_3D('',#36932,#28763,#28764);
#24619=AXIS2_PLACEMENT_3D('',#36956,#28766,#28767);
#24620=AXIS2_PLACEMENT_3D('',#36981,#28769,#28770);
#24621=AXIS2_PLACEMENT_3D('',#37006,#28772,#28773);
#24622=AXIS2_PLACEMENT_3D('',#37030,#28775,#28776);
#24623=AXIS2_PLACEMENT_3D('',#37055,#28778,#28779);
#24624=AXIS2_PLACEMENT_3D('',#37080,#28781,#28782);
#24625=AXIS2_PLACEMENT_3D('',#37104,#28784,#28785);
#24626=AXIS2_PLACEMENT_3D('',#37128,#28787,#28788);
#24627=AXIS2_PLACEMENT_3D('',#37153,#28790,#28791);
#24628=AXIS2_PLACEMENT_3D('',#37178,#28793,#28794);
#24629=AXIS2_PLACEMENT_3D('',#37183,#28796,#28797);
#24630=AXIS2_PLACEMENT_3D('',#37712,#28798,#28799);
#24631=AXIS2_PLACEMENT_3D('',#37765,#28800,#28801);
#24632=AXIS2_PLACEMENT_3D('',#37766,#28802,#28803);
#24633=AXIS2_PLACEMENT_3D('',#38216,#28804,#28805);
#24634=AXIS2_PLACEMENT_3D('',#38217,#28806,#28807);
#24635=AXIS2_PLACEMENT_3D('',#38218,#28808,#28809);
#24636=AXIS2_PLACEMENT_3D('',#38222,#28811,#28812);
#24637=AXIS2_PLACEMENT_3D('',#38223,#28813,#28814);
#24638=AXIS2_PLACEMENT_3D('',#38232,#28819,#28820);
#24639=AXIS2_PLACEMENT_3D('',#38234,#28821,#28822);
#24640=AXIS2_PLACEMENT_3D('',#38236,#28824,#28825);
#24641=AXIS2_PLACEMENT_3D('',#38240,#28828,#28829);
#24642=AXIS2_PLACEMENT_3D('',#38241,#28830,#28831);
#24643=AXIS2_PLACEMENT_3D('',#38242,#28832,#28833);
#24644=AXIS2_PLACEMENT_3D('',#38251,#28838,#28839);
#24645=AXIS2_PLACEMENT_3D('',#38253,#28840,#28841);
#24646=AXIS2_PLACEMENT_3D('',#38255,#28843,#28844);
#24647=AXIS2_PLACEMENT_3D('',#38259,#28847,#28848);
#24648=AXIS2_PLACEMENT_3D('',#38260,#28849,#28850);
#24649=AXIS2_PLACEMENT_3D('',#38261,#28851,#28852);
#24650=AXIS2_PLACEMENT_3D('',#38270,#28857,#28858);
#24651=AXIS2_PLACEMENT_3D('',#38272,#28859,#28860);
#24652=AXIS2_PLACEMENT_3D('',#38274,#28862,#28863);
#24653=AXIS2_PLACEMENT_3D('',#38278,#28866,#28867);
#24654=AXIS2_PLACEMENT_3D('',#38279,#28868,#28869);
#24655=AXIS2_PLACEMENT_3D('',#38280,#28870,#28871);
#24656=AXIS2_PLACEMENT_3D('',#38289,#28876,#28877);
#24657=AXIS2_PLACEMENT_3D('',#38291,#28878,#28879);
#24658=AXIS2_PLACEMENT_3D('',#38293,#28881,#28882);
#24659=AXIS2_PLACEMENT_3D('',#38297,#28885,#28886);
#24660=AXIS2_PLACEMENT_3D('',#38298,#28887,#28888);
#24661=AXIS2_PLACEMENT_3D('',#38299,#28889,#28890);
#24662=AXIS2_PLACEMENT_3D('',#38308,#28895,#28896);
#24663=AXIS2_PLACEMENT_3D('',#38310,#28897,#28898);
#24664=AXIS2_PLACEMENT_3D('',#38312,#28900,#28901);
#24665=AXIS2_PLACEMENT_3D('',#38316,#28904,#28905);
#24666=AXIS2_PLACEMENT_3D('',#38317,#28906,#28907);
#24667=AXIS2_PLACEMENT_3D('',#38318,#28908,#28909);
#24668=AXIS2_PLACEMENT_3D('',#38327,#28914,#28915);
#24669=AXIS2_PLACEMENT_3D('',#38329,#28916,#28917);
#24670=AXIS2_PLACEMENT_3D('',#38331,#28919,#28920);
#24671=AXIS2_PLACEMENT_3D('',#38335,#28923,#28924);
#24672=AXIS2_PLACEMENT_3D('',#38336,#28925,#28926);
#24673=AXIS2_PLACEMENT_3D('',#38337,#28927,#28928);
#24674=AXIS2_PLACEMENT_3D('',#38346,#28933,#28934);
#24675=AXIS2_PLACEMENT_3D('',#38348,#28935,#28936);
#24676=AXIS2_PLACEMENT_3D('',#38350,#28938,#28939);
#24677=AXIS2_PLACEMENT_3D('',#38354,#28942,#28943);
#24678=AXIS2_PLACEMENT_3D('',#38355,#28944,#28945);
#24679=AXIS2_PLACEMENT_3D('',#38356,#28946,#28947);
#24680=AXIS2_PLACEMENT_3D('',#38365,#28952,#28953);
#24681=AXIS2_PLACEMENT_3D('',#38367,#28954,#28955);
#24682=AXIS2_PLACEMENT_3D('',#38369,#28957,#28958);
#24683=AXIS2_PLACEMENT_3D('',#38373,#28961,#28962);
#24684=AXIS2_PLACEMENT_3D('',#38374,#28963,#28964);
#24685=AXIS2_PLACEMENT_3D('',#38375,#28965,#28966);
#24686=AXIS2_PLACEMENT_3D('',#38384,#28971,#28972);
#24687=AXIS2_PLACEMENT_3D('',#38386,#28973,#28974);
#24688=AXIS2_PLACEMENT_3D('',#38388,#28976,#28977);
#24689=AXIS2_PLACEMENT_3D('',#38392,#28980,#28981);
#24690=AXIS2_PLACEMENT_3D('',#38393,#28982,#28983);
#24691=AXIS2_PLACEMENT_3D('',#38394,#28984,#28985);
#24692=AXIS2_PLACEMENT_3D('',#38403,#28990,#28991);
#24693=AXIS2_PLACEMENT_3D('',#38405,#28992,#28993);
#24694=AXIS2_PLACEMENT_3D('',#38407,#28995,#28996);
#24695=AXIS2_PLACEMENT_3D('',#38411,#28999,#29000);
#24696=AXIS2_PLACEMENT_3D('',#38412,#29001,#29002);
#24697=AXIS2_PLACEMENT_3D('',#38413,#29003,#29004);
#24698=AXIS2_PLACEMENT_3D('',#38422,#29009,#29010);
#24699=AXIS2_PLACEMENT_3D('',#38424,#29011,#29012);
#24700=AXIS2_PLACEMENT_3D('',#38426,#29014,#29015);
#24701=AXIS2_PLACEMENT_3D('',#38430,#29018,#29019);
#24702=AXIS2_PLACEMENT_3D('',#38431,#29020,#29021);
#24703=AXIS2_PLACEMENT_3D('',#38432,#29022,#29023);
#24704=AXIS2_PLACEMENT_3D('',#38441,#29028,#29029);
#24705=AXIS2_PLACEMENT_3D('',#38443,#29030,#29031);
#24706=AXIS2_PLACEMENT_3D('',#38446,#29033,#29034);
#24707=AXIS2_PLACEMENT_3D('',#38447,#29035,#29036);
#24708=AXIS2_PLACEMENT_3D('',#38451,#29039,#29040);
#24709=AXIS2_PLACEMENT_3D('',#38453,#29041,#29042);
#24710=AXIS2_PLACEMENT_3D('',#38454,#29043,#29044);
#24711=AXIS2_PLACEMENT_3D('',#38455,#29045,#29046);
#24712=AXIS2_PLACEMENT_3D('',#38464,#29051,#29052);
#24713=AXIS2_PLACEMENT_3D('',#38466,#29053,#29054);
#24714=AXIS2_PLACEMENT_3D('',#38468,#29056,#29057);
#24715=AXIS2_PLACEMENT_3D('',#38472,#29060,#29061);
#24716=AXIS2_PLACEMENT_3D('',#38473,#29062,#29063);
#24717=AXIS2_PLACEMENT_3D('',#38474,#29064,#29065);
#24718=AXIS2_PLACEMENT_3D('',#38483,#29070,#29071);
#24719=AXIS2_PLACEMENT_3D('',#38485,#29072,#29073);
#24720=AXIS2_PLACEMENT_3D('',#38487,#29075,#29076);
#24721=AXIS2_PLACEMENT_3D('',#38491,#29079,#29080);
#24722=AXIS2_PLACEMENT_3D('',#38492,#29081,#29082);
#24723=AXIS2_PLACEMENT_3D('',#38493,#29083,#29084);
#24724=AXIS2_PLACEMENT_3D('',#38502,#29089,#29090);
#24725=AXIS2_PLACEMENT_3D('',#38504,#29091,#29092);
#24726=AXIS2_PLACEMENT_3D('',#38506,#29094,#29095);
#24727=AXIS2_PLACEMENT_3D('',#38510,#29098,#29099);
#24728=AXIS2_PLACEMENT_3D('',#38511,#29100,#29101);
#24729=AXIS2_PLACEMENT_3D('',#38512,#29102,#29103);
#24730=AXIS2_PLACEMENT_3D('',#38521,#29108,#29109);
#24731=AXIS2_PLACEMENT_3D('',#38523,#29110,#29111);
#24732=AXIS2_PLACEMENT_3D('',#38525,#29113,#29114);
#24733=AXIS2_PLACEMENT_3D('',#38529,#29117,#29118);
#24734=AXIS2_PLACEMENT_3D('',#38530,#29119,#29120);
#24735=AXIS2_PLACEMENT_3D('',#38531,#29121,#29122);
#24736=AXIS2_PLACEMENT_3D('',#38540,#29127,#29128);
#24737=AXIS2_PLACEMENT_3D('',#38542,#29129,#29130);
#24738=AXIS2_PLACEMENT_3D('',#38544,#29132,#29133);
#24739=AXIS2_PLACEMENT_3D('',#38548,#29136,#29137);
#24740=AXIS2_PLACEMENT_3D('',#38549,#29138,#29139);
#24741=AXIS2_PLACEMENT_3D('',#38550,#29140,#29141);
#24742=AXIS2_PLACEMENT_3D('',#38559,#29146,#29147);
#24743=AXIS2_PLACEMENT_3D('',#38561,#29148,#29149);
#24744=AXIS2_PLACEMENT_3D('',#38563,#29151,#29152);
#24745=AXIS2_PLACEMENT_3D('',#38567,#29155,#29156);
#24746=AXIS2_PLACEMENT_3D('',#38568,#29157,#29158);
#24747=AXIS2_PLACEMENT_3D('',#38569,#29159,#29160);
#24748=AXIS2_PLACEMENT_3D('',#38578,#29165,#29166);
#24749=AXIS2_PLACEMENT_3D('',#38580,#29167,#29168);
#24750=AXIS2_PLACEMENT_3D('',#38582,#29170,#29171);
#24751=AXIS2_PLACEMENT_3D('',#38586,#29174,#29175);
#24752=AXIS2_PLACEMENT_3D('',#38587,#29176,#29177);
#24753=AXIS2_PLACEMENT_3D('',#38588,#29178,#29179);
#24754=AXIS2_PLACEMENT_3D('',#38597,#29184,#29185);
#24755=AXIS2_PLACEMENT_3D('',#38599,#29186,#29187);
#24756=AXIS2_PLACEMENT_3D('',#38601,#29189,#29190);
#24757=AXIS2_PLACEMENT_3D('',#38605,#29193,#29194);
#24758=AXIS2_PLACEMENT_3D('',#38606,#29195,#29196);
#24759=AXIS2_PLACEMENT_3D('',#38607,#29197,#29198);
#24760=AXIS2_PLACEMENT_3D('',#38616,#29203,#29204);
#24761=AXIS2_PLACEMENT_3D('',#38618,#29205,#29206);
#24762=AXIS2_PLACEMENT_3D('',#38620,#29208,#29209);
#24763=AXIS2_PLACEMENT_3D('',#38624,#29212,#29213);
#24764=AXIS2_PLACEMENT_3D('',#38625,#29214,#29215);
#24765=AXIS2_PLACEMENT_3D('',#38626,#29216,#29217);
#24766=AXIS2_PLACEMENT_3D('',#38635,#29222,#29223);
#24767=AXIS2_PLACEMENT_3D('',#38637,#29224,#29225);
#24768=AXIS2_PLACEMENT_3D('',#38639,#29227,#29228);
#24769=AXIS2_PLACEMENT_3D('',#38643,#29231,#29232);
#24770=AXIS2_PLACEMENT_3D('',#38644,#29233,#29234);
#24771=AXIS2_PLACEMENT_3D('',#38645,#29235,#29236);
#24772=AXIS2_PLACEMENT_3D('',#38654,#29241,#29242);
#24773=AXIS2_PLACEMENT_3D('',#38656,#29243,#29244);
#24774=AXIS2_PLACEMENT_3D('',#38658,#29246,#29247);
#24775=AXIS2_PLACEMENT_3D('',#38662,#29250,#29251);
#24776=AXIS2_PLACEMENT_3D('',#38663,#29252,#29253);
#24777=AXIS2_PLACEMENT_3D('',#38664,#29254,#29255);
#24778=AXIS2_PLACEMENT_3D('',#38673,#29260,#29261);
#24779=AXIS2_PLACEMENT_3D('',#38675,#29262,#29263);
#24780=AXIS2_PLACEMENT_3D('',#38677,#29265,#29266);
#24781=AXIS2_PLACEMENT_3D('',#38681,#29269,#29270);
#24782=AXIS2_PLACEMENT_3D('',#38682,#29271,#29272);
#24783=AXIS2_PLACEMENT_3D('',#38683,#29273,#29274);
#24784=AXIS2_PLACEMENT_3D('',#38685,#29275,#29276);
#24785=AXIS2_PLACEMENT_3D('',#38686,#29277,#29278);
#24786=AXIS2_PLACEMENT_3D('',#38688,#29280,#29281);
#24787=AXIS2_PLACEMENT_3D('',#38690,#29282,#29283);
#24788=AXIS2_PLACEMENT_3D('',#38691,#29284,#29285);
#24789=AXIS2_PLACEMENT_3D('',#38693,#29286,#29287);
#24790=AXIS2_PLACEMENT_3D('',#38695,#29289,#29290);
#24791=AXIS2_PLACEMENT_3D('',#38697,#29291,#29292);
#24792=AXIS2_PLACEMENT_3D('',#38700,#29295,#29296);
#24793=AXIS2_PLACEMENT_3D('',#38702,#29297,#29298);
#24794=AXIS2_PLACEMENT_3D('',#38704,#29300,#29301);
#28698=DIRECTION('axis',(0.,0.,1.));
#28699=DIRECTION('refdir',(1.,0.,0.));
#28700=DIRECTION('center_axis',(0.,0.,1.));
#28701=DIRECTION('ref_axis',(1.,0.,0.));
#28702=DIRECTION('',(0.,0.,-1.));
#28703=DIRECTION('center_axis',(0.,0.,-1.));
#28704=DIRECTION('ref_axis',(1.,0.,0.));
#28705=DIRECTION('',(0.,0.,-1.));
#28706=DIRECTION('center_axis',(0.,0.,1.));
#28707=DIRECTION('ref_axis',(1.,0.,0.));
#28708=DIRECTION('center_axis',(0.,0.,-1.));
#28709=DIRECTION('ref_axis',(1.,0.,0.));
#28710=DIRECTION('center_axis',(0.,0.,1.));
#28711=DIRECTION('ref_axis',(1.,0.,0.));
#28712=DIRECTION('',(0.,0.,-1.));
#28713=DIRECTION('center_axis',(0.,0.,1.));
#28714=DIRECTION('ref_axis',(1.,0.,0.));
#28715=DIRECTION('',(0.,0.,-1.));
#28716=DIRECTION('center_axis',(0.,0.,1.));
#28717=DIRECTION('ref_axis',(1.,0.,0.));
#28718=DIRECTION('',(0.,0.,-1.));
#28719=DIRECTION('center_axis',(0.,0.,1.));
#28720=DIRECTION('ref_axis',(1.,0.,0.));
#28721=DIRECTION('',(0.,0.,-1.));
#28722=DIRECTION('center_axis',(0.,0.,1.));
#28723=DIRECTION('ref_axis',(1.,0.,0.));
#28724=DIRECTION('',(0.,0.,-1.));
#28725=DIRECTION('center_axis',(0.,0.,1.));
#28726=DIRECTION('ref_axis',(1.,0.,0.));
#28727=DIRECTION('',(0.,0.,-1.));
#28728=DIRECTION('center_axis',(0.,0.,1.));
#28729=DIRECTION('ref_axis',(1.,0.,0.));
#28730=DIRECTION('',(0.,0.,-1.));
#28731=DIRECTION('center_axis',(0.,0.,1.));
#28732=DIRECTION('ref_axis',(1.,0.,0.));
#28733=DIRECTION('',(0.,0.,-1.));
#28734=DIRECTION('center_axis',(0.,0.,1.));
#28735=DIRECTION('ref_axis',(1.,0.,0.));
#28736=DIRECTION('',(0.,0.,-1.));
#28737=DIRECTION('center_axis',(0.,0.,1.));
#28738=DIRECTION('ref_axis',(1.,0.,0.));
#28739=DIRECTION('',(0.,0.,-1.));
#28740=DIRECTION('center_axis',(0.,0.,1.));
#28741=DIRECTION('ref_axis',(1.,0.,0.));
#28742=DIRECTION('',(0.,0.,-1.));
#28743=DIRECTION('center_axis',(0.,0.,1.));
#28744=DIRECTION('ref_axis',(1.,0.,0.));
#28745=DIRECTION('',(0.,0.,-1.));
#28746=DIRECTION('center_axis',(0.,0.,1.));
#28747=DIRECTION('ref_axis',(1.,0.,0.));
#28748=DIRECTION('',(0.,0.,-1.));
#28749=DIRECTION('center_axis',(0.,0.,1.));
#28750=DIRECTION('ref_axis',(-0.266010203854043,-0.963970212945157,0.));
#28751=DIRECTION('',(0.,0.,1.));
#28752=DIRECTION('center_axis',(0.,0.,1.));
#28753=DIRECTION('ref_axis',(1.,8.51023079448757E-14,0.));
#28754=DIRECTION('center_axis',(0.,0.,1.));
#28755=DIRECTION('ref_axis',(1.,8.51023079448757E-14,0.));
#28756=DIRECTION('',(0.,0.,1.));
#28757=DIRECTION('center_axis',(0.,0.,1.));
#28758=DIRECTION('ref_axis',(1.,8.51023079448757E-14,0.));
#28759=DIRECTION('',(0.,0.,1.));
#28760=DIRECTION('center_axis',(0.,0.,1.));
#28761=DIRECTION('ref_axis',(1.,8.51023079448757E-14,0.));
#28762=DIRECTION('',(0.,0.,1.));
#28763=DIRECTION('center_axis',(0.,0.,1.));
#28764=DIRECTION('ref_axis',(1.,8.51023079448757E-14,0.));
#28765=DIRECTION('',(0.,0.,1.));
#28766=DIRECTION('center_axis',(0.,0.,1.));
#28767=DIRECTION('ref_axis',(1.,8.51023079448757E-14,0.));
#28768=DIRECTION('',(0.,0.,1.));
#28769=DIRECTION('center_axis',(0.,0.,1.));
#28770=DIRECTION('ref_axis',(1.,8.51023079448757E-14,0.));
#28771=DIRECTION('',(0.,0.,1.));
#28772=DIRECTION('center_axis',(0.,0.,1.));
#28773=DIRECTION('ref_axis',(1.,8.51023079448757E-14,0.));
#28774=DIRECTION('',(0.,0.,1.));
#28775=DIRECTION('center_axis',(0.,0.,1.));
#28776=DIRECTION('ref_axis',(1.,8.51023079448757E-14,0.));
#28777=DIRECTION('',(0.,0.,1.));
#28778=DIRECTION('center_axis',(0.,0.,1.));
#28779=DIRECTION('ref_axis',(1.,8.51023079448757E-14,0.));
#28780=DIRECTION('',(0.,0.,1.));
#28781=DIRECTION('center_axis',(0.,0.,1.));
#28782=DIRECTION('ref_axis',(1.,8.51023079448757E-14,0.));
#28783=DIRECTION('',(0.,0.,1.));
#28784=DIRECTION('center_axis',(0.,0.,1.));
#28785=DIRECTION('ref_axis',(1.,8.51023079448757E-14,0.));
#28786=DIRECTION('',(0.,0.,1.));
#28787=DIRECTION('center_axis',(0.,0.,1.));
#28788=DIRECTION('ref_axis',(1.,8.51023079448757E-14,0.));
#28789=DIRECTION('',(0.,0.,1.));
#28790=DIRECTION('center_axis',(0.,0.,1.));
#28791=DIRECTION('ref_axis',(1.,8.51023079448757E-14,0.));
#28792=DIRECTION('',(0.,0.,1.));
#28793=DIRECTION('center_axis',(0.,0.,1.));
#28794=DIRECTION('ref_axis',(1.,8.51023079448757E-14,0.));
#28795=DIRECTION('',(0.,0.,1.));
#28796=DIRECTION('center_axis',(0.,0.,-1.));
#28797=DIRECTION('ref_axis',(1.,8.51023079448757E-14,0.));
#28798=DIRECTION('center_axis',(0.,0.,1.));
#28799=DIRECTION('ref_axis',(1.,0.,0.));
#28800=DIRECTION('center_axis',(0.,0.,-1.));
#28801=DIRECTION('ref_axis',(1.,8.51023079448757E-14,0.));
#28802=DIRECTION('center_axis',(0.,0.,1.));
#28803=DIRECTION('ref_axis',(1.,8.51023079448757E-14,0.));
#28804=DIRECTION('center_axis',(0.,0.,1.));
#28805=DIRECTION('ref_axis',(0.939073080792118,-0.343717542368148,0.));
#28806=DIRECTION('center_axis',(0.,0.,1.));
#28807=DIRECTION('ref_axis',(1.,0.,0.));
#28808=DIRECTION('center_axis',(0.,0.,1.));
#28809=DIRECTION('ref_axis',(1.,0.,0.));
#28810=DIRECTION('',(-0.957826285221151,-1.17299889433528E-16,0.287347885566345));
#28811=DIRECTION('center_axis',(0.,0.,-1.));
#28812=DIRECTION('ref_axis',(1.,0.,0.));
#28813=DIRECTION('center_axis',(-0.706367935150259,-0.707844856018294,0.));
#28814=DIRECTION('ref_axis',(0.707844856018294,-0.706367935150259,0.));
#28815=DIRECTION('',(0.,0.,1.));
#28816=DIRECTION('',(0.707844856018294,-0.706367935150259,0.));
#28817=DIRECTION('',(0.,0.,1.));
#28818=DIRECTION('',(0.707844856018294,-0.706367935150259,0.));
#28819=DIRECTION('center_axis',(0.,0.,1.));
#28820=DIRECTION('ref_axis',(0.965925826289068,-0.258819045102522,0.));
#28821=DIRECTION('center_axis',(0.,0.,1.));
#28822=DIRECTION('ref_axis',(1.,0.,0.));
#28823=DIRECTION('',(-0.966195594825111,-0.257810148249735,0.));
#28824=DIRECTION('center_axis',(-0.257810148249735,0.966195594825111,0.));
#28825=DIRECTION('ref_axis',(-0.966195594825111,-0.257810148249735,0.));
#28826=DIRECTION('',(0.,0.,-1.));
#28827=DIRECTION('',(-0.966195594825111,-0.257810148249735,0.));
#28828=DIRECTION('center_axis',(0.,0.,1.));
#28829=DIRECTION('ref_axis',(0.965925826289068,-0.258819045102522,0.));
#28830=DIRECTION('center_axis',(0.,0.,-1.));
#28831=DIRECTION('ref_axis',(1.,0.,0.));
#28832=DIRECTION('center_axis',(-0.865502761139503,-0.500904152967308,0.));
#28833=DIRECTION('ref_axis',(0.500904152967308,-0.865502761139503,0.));
#28834=DIRECTION('',(0.,0.,1.));
#28835=DIRECTION('',(0.500904152967308,-0.865502761139503,0.));
#28836=DIRECTION('',(0.,0.,1.));
#28837=DIRECTION('',(0.500904152967308,-0.865502761139503,0.));
#28838=DIRECTION('center_axis',(0.,0.,1.));
#28839=DIRECTION('ref_axis',(0.866025403784438,-0.500000000000001,0.));
#28840=DIRECTION('center_axis',(0.,0.,1.));
#28841=DIRECTION('ref_axis',(1.,0.,0.));
#28842=DIRECTION('',(-0.999999454676039,0.00104434076106441,0.));
#28843=DIRECTION('center_axis',(0.00104434076106438,0.999999454676039,0.));
#28844=DIRECTION('ref_axis',(-0.999999454676039,0.00104434076106438,0.));
#28845=DIRECTION('',(0.,0.,-1.));
#28846=DIRECTION('',(-0.999999454676039,0.00104434076106441,0.));
#28847=DIRECTION('center_axis',(0.,0.,1.));
#28848=DIRECTION('ref_axis',(0.866025403784438,-0.500000000000001,0.));
#28849=DIRECTION('center_axis',(0.,0.,-1.));
#28850=DIRECTION('ref_axis',(1.,0.,0.));
#28851=DIRECTION('center_axis',(-0.96565500426803,-0.259827659674851,0.));
#28852=DIRECTION('ref_axis',(0.259827659674851,-0.96565500426803,0.));
#28853=DIRECTION('',(0.,0.,1.));
#28854=DIRECTION('',(0.259827659674851,-0.96565500426803,0.));
#28855=DIRECTION('',(0.,0.,1.));
#28856=DIRECTION('',(0.259827659674851,-0.96565500426803,0.));
#28857=DIRECTION('center_axis',(0.,0.,1.));
#28858=DIRECTION('ref_axis',(0.707106781186547,-0.707106781186548,0.));
#28859=DIRECTION('center_axis',(0.,0.,1.));
#28860=DIRECTION('ref_axis',(1.,0.,0.));
#28861=DIRECTION('',(-0.96565500426803,0.259827659674852,0.));
#28862=DIRECTION('center_axis',(0.259827659674852,0.96565500426803,0.));
#28863=DIRECTION('ref_axis',(-0.96565500426803,0.259827659674852,0.));
#28864=DIRECTION('',(0.,0.,-1.));
#28865=DIRECTION('',(-0.96565500426803,0.259827659674852,0.));
#28866=DIRECTION('center_axis',(0.,0.,1.));
#28867=DIRECTION('ref_axis',(0.707106781186547,-0.707106781186548,0.));
#28868=DIRECTION('center_axis',(0.,0.,-1.));
#28869=DIRECTION('ref_axis',(1.,0.,0.));
#28870=DIRECTION('center_axis',(-0.999999454676039,-0.00104434076106302,
0.));
#28871=DIRECTION('ref_axis',(0.00104434076106302,-0.999999454676039,0.));
#28872=DIRECTION('',(0.,0.,1.));
#28873=DIRECTION('',(0.00104434076106297,-0.999999454676039,0.));
#28874=DIRECTION('',(0.,0.,1.));
#28875=DIRECTION('',(0.00104434076106297,-0.999999454676039,0.));
#28876=DIRECTION('center_axis',(0.,0.,1.));
#28877=DIRECTION('ref_axis',(0.499999999999999,-0.866025403784439,0.));
#28878=DIRECTION('center_axis',(0.,0.,1.));
#28879=DIRECTION('ref_axis',(1.,0.,0.));
#28880=DIRECTION('',(-0.865502761139503,0.500904152967309,0.));
#28881=DIRECTION('center_axis',(0.500904152967309,0.865502761139503,0.));
#28882=DIRECTION('ref_axis',(-0.865502761139503,0.500904152967309,0.));
#28883=DIRECTION('',(0.,0.,-1.));
#28884=DIRECTION('',(-0.865502761139503,0.500904152967309,0.));
#28885=DIRECTION('center_axis',(0.,0.,1.));
#28886=DIRECTION('ref_axis',(0.499999999999999,-0.866025403784439,0.));
#28887=DIRECTION('center_axis',(0.,0.,-1.));
#28888=DIRECTION('ref_axis',(1.,0.,0.));
#28889=DIRECTION('center_axis',(-0.966195594825111,0.257810148249736,0.));
#28890=DIRECTION('ref_axis',(-0.257810148249736,-0.966195594825111,0.));
#28891=DIRECTION('',(0.,0.,1.));
#28892=DIRECTION('',(-0.257810148249736,-0.96619559482511,0.));
#28893=DIRECTION('',(0.,0.,1.));
#28894=DIRECTION('',(-0.257810148249736,-0.96619559482511,0.));
#28895=DIRECTION('center_axis',(0.,0.,1.));
#28896=DIRECTION('ref_axis',(0.25881904510252,-0.965925826289068,0.));
#28897=DIRECTION('center_axis',(0.,0.,1.));
#28898=DIRECTION('ref_axis',(1.,0.,0.));
#28899=DIRECTION('',(-0.706367935150259,0.707844856018295,0.));
#28900=DIRECTION('center_axis',(0.707844856018295,0.706367935150259,0.));
#28901=DIRECTION('ref_axis',(-0.706367935150259,0.707844856018295,0.));
#28902=DIRECTION('',(0.,0.,-1.));
#28903=DIRECTION('',(-0.706367935150259,0.707844856018295,0.));
#28904=DIRECTION('center_axis',(0.,0.,1.));
#28905=DIRECTION('ref_axis',(0.25881904510252,-0.965925826289068,0.));
#28906=DIRECTION('center_axis',(0.,0.,-1.));
#28907=DIRECTION('ref_axis',(1.,0.,0.));
#28908=DIRECTION('center_axis',(-0.866547101900567,0.499095301708731,0.));
#28909=DIRECTION('ref_axis',(-0.499095301708731,-0.866547101900567,0.));
#28910=DIRECTION('',(0.,0.,1.));
#28911=DIRECTION('',(-0.499095301708731,-0.866547101900567,0.));
#28912=DIRECTION('',(0.,0.,1.));
#28913=DIRECTION('',(-0.499095301708731,-0.866547101900567,0.));
#28914=DIRECTION('center_axis',(0.,0.,1.));
#28915=DIRECTION('ref_axis',(-1.94289029309402E-16,-1.,0.));
#28916=DIRECTION('center_axis',(0.,0.,1.));
#28917=DIRECTION('ref_axis',(1.,0.,0.));
#28918=DIRECTION('',(-0.49909530170873,0.866547101900567,0.));
#28919=DIRECTION('center_axis',(0.866547101900567,0.49909530170873,0.));
#28920=DIRECTION('ref_axis',(-0.49909530170873,0.866547101900567,0.));
#28921=DIRECTION('',(0.,0.,-1.));
#28922=DIRECTION('',(-0.49909530170873,0.866547101900567,0.));
#28923=DIRECTION('center_axis',(0.,0.,1.));
#28924=DIRECTION('ref_axis',(-1.94289029309402E-16,-1.,0.));
#28925=DIRECTION('center_axis',(0.,0.,-1.));
#28926=DIRECTION('ref_axis',(1.,0.,0.));
#28927=DIRECTION('center_axis',(-0.707844856018294,0.706367935150259,0.));
#28928=DIRECTION('ref_axis',(-0.706367935150259,-0.707844856018294,0.));
#28929=DIRECTION('',(0.,0.,1.));
#28930=DIRECTION('',(-0.706367935150259,-0.707844856018294,0.));
#28931=DIRECTION('',(0.,0.,1.));
#28932=DIRECTION('',(-0.706367935150259,-0.707844856018294,0.));
#28933=DIRECTION('center_axis',(0.,0.,1.));
#28934=DIRECTION('ref_axis',(-0.258819045102522,-0.965925826289068,0.));
#28935=DIRECTION('center_axis',(0.,0.,1.));
#28936=DIRECTION('ref_axis',(1.,0.,0.));
#28937=DIRECTION('',(-0.257810148249735,0.966195594825111,0.));
#28938=DIRECTION('center_axis',(0.966195594825111,0.257810148249735,0.));
#28939=DIRECTION('ref_axis',(-0.257810148249735,0.966195594825111,0.));
#28940=DIRECTION('',(0.,0.,-1.));
#28941=DIRECTION('',(-0.257810148249735,0.966195594825111,0.));
#28942=DIRECTION('center_axis',(0.,0.,1.));
#28943=DIRECTION('ref_axis',(-0.258819045102522,-0.965925826289068,0.));
#28944=DIRECTION('center_axis',(0.,0.,-1.));
#28945=DIRECTION('ref_axis',(1.,0.,0.));
#28946=DIRECTION('center_axis',(-0.500904152967308,0.865502761139503,0.));
#28947=DIRECTION('ref_axis',(-0.865502761139503,-0.500904152967308,0.));
#28948=DIRECTION('',(0.,0.,1.));
#28949=DIRECTION('',(-0.865502761139503,-0.500904152967308,0.));
#28950=DIRECTION('',(0.,0.,1.));
#28951=DIRECTION('',(-0.865502761139503,-0.500904152967308,0.));
#28952=DIRECTION('center_axis',(0.,0.,1.));
#28953=DIRECTION('ref_axis',(-0.500000000000001,-0.866025403784438,0.));
#28954=DIRECTION('center_axis',(0.,0.,1.));
#28955=DIRECTION('ref_axis',(1.,0.,0.));
#28956=DIRECTION('',(0.00104434076106441,0.999999454676039,0.));
#28957=DIRECTION('center_axis',(0.999999454676039,-0.00104434076106438,
0.));
#28958=DIRECTION('ref_axis',(0.00104434076106438,0.999999454676039,0.));
#28959=DIRECTION('',(0.,0.,-1.));
#28960=DIRECTION('',(0.00104434076106441,0.999999454676039,0.));
#28961=DIRECTION('center_axis',(0.,0.,1.));
#28962=DIRECTION('ref_axis',(-0.500000000000001,-0.866025403784438,0.));
#28963=DIRECTION('center_axis',(0.,0.,-1.));
#28964=DIRECTION('ref_axis',(1.,0.,0.));
#28965=DIRECTION('center_axis',(-0.259827659674851,0.96565500426803,0.));
#28966=DIRECTION('ref_axis',(-0.96565500426803,-0.259827659674851,0.));
#28967=DIRECTION('',(0.,0.,1.));
#28968=DIRECTION('',(-0.96565500426803,-0.259827659674851,0.));
#28969=DIRECTION('',(0.,0.,1.));
#28970=DIRECTION('',(-0.96565500426803,-0.259827659674851,0.));
#28971=DIRECTION('center_axis',(0.,0.,1.));
#28972=DIRECTION('ref_axis',(-0.707106781186548,-0.707106781186547,0.));
#28973=DIRECTION('center_axis',(0.,0.,1.));
#28974=DIRECTION('ref_axis',(1.,0.,0.));
#28975=DIRECTION('',(0.259827659674852,0.96565500426803,0.));
#28976=DIRECTION('center_axis',(0.96565500426803,-0.259827659674852,0.));
#28977=DIRECTION('ref_axis',(0.259827659674852,0.96565500426803,0.));
#28978=DIRECTION('',(0.,0.,-1.));
#28979=DIRECTION('',(0.259827659674852,0.96565500426803,0.));
#28980=DIRECTION('center_axis',(0.,0.,1.));
#28981=DIRECTION('ref_axis',(-0.707106781186548,-0.707106781186547,0.));
#28982=DIRECTION('center_axis',(0.,0.,-1.));
#28983=DIRECTION('ref_axis',(1.,0.,0.));
#28984=DIRECTION('center_axis',(-0.00104434076106344,0.999999454676039,
0.));
#28985=DIRECTION('ref_axis',(-0.999999454676039,-0.00104434076106344,0.));
#28986=DIRECTION('',(0.,0.,1.));
#28987=DIRECTION('',(-0.999999454676039,-0.00104434076106344,0.));
#28988=DIRECTION('',(0.,0.,1.));
#28989=DIRECTION('',(-0.999999454676039,-0.00104434076106344,0.));
#28990=DIRECTION('center_axis',(0.,0.,1.));
#28991=DIRECTION('ref_axis',(-0.866025403784439,-0.5,0.));
#28992=DIRECTION('center_axis',(0.,0.,1.));
#28993=DIRECTION('ref_axis',(1.,0.,0.));
#28994=DIRECTION('',(0.500904152967309,0.865502761139503,0.));
#28995=DIRECTION('center_axis',(0.865502761139503,-0.500904152967309,0.));
#28996=DIRECTION('ref_axis',(0.500904152967309,0.865502761139503,0.));
#28997=DIRECTION('',(0.,0.,-1.));
#28998=DIRECTION('',(0.500904152967309,0.865502761139503,0.));
#28999=DIRECTION('center_axis',(0.,0.,1.));
#29000=DIRECTION('ref_axis',(-0.866025403784439,-0.5,0.));
#29001=DIRECTION('center_axis',(0.,0.,-1.));
#29002=DIRECTION('ref_axis',(1.,0.,0.));
#29003=DIRECTION('center_axis',(0.257810148249736,0.966195594825111,0.));
#29004=DIRECTION('ref_axis',(-0.966195594825111,0.257810148249736,0.));
#29005=DIRECTION('',(0.,0.,1.));
#29006=DIRECTION('',(-0.96619559482511,0.257810148249736,0.));
#29007=DIRECTION('',(0.,0.,1.));
#29008=DIRECTION('',(-0.96619559482511,0.257810148249736,0.));
#29009=DIRECTION('center_axis',(0.,0.,1.));
#29010=DIRECTION('ref_axis',(-0.965925826289068,-0.25881904510252,0.));
#29011=DIRECTION('center_axis',(0.,0.,1.));
#29012=DIRECTION('ref_axis',(1.,0.,0.));
#29013=DIRECTION('',(0.707844856018295,0.706367935150259,0.));
#29014=DIRECTION('center_axis',(0.706367935150259,-0.707844856018295,0.));
#29015=DIRECTION('ref_axis',(0.707844856018295,0.706367935150259,0.));
#29016=DIRECTION('',(0.,0.,-1.));
#29017=DIRECTION('',(0.707844856018295,0.706367935150259,0.));
#29018=DIRECTION('center_axis',(0.,0.,1.));
#29019=DIRECTION('ref_axis',(-0.965925826289068,-0.25881904510252,0.));
#29020=DIRECTION('center_axis',(0.,0.,-1.));
#29021=DIRECTION('ref_axis',(1.,0.,0.));
#29022=DIRECTION('center_axis',(0.499095301708731,0.866547101900567,0.));
#29023=DIRECTION('ref_axis',(-0.866547101900567,0.499095301708731,0.));
#29024=DIRECTION('',(0.,0.,1.));
#29025=DIRECTION('',(-0.866547101900567,0.499095301708731,0.));
#29026=DIRECTION('',(0.,0.,1.));
#29027=DIRECTION('',(-0.866547101900567,0.499095301708731,0.));
#29028=DIRECTION('center_axis',(0.,0.,1.));
#29029=DIRECTION('ref_axis',(-1.,1.38777878078145E-16,0.));
#29030=DIRECTION('center_axis',(0.,0.,1.));
#29031=DIRECTION('ref_axis',(1.,0.,0.));
#29032=DIRECTION('',(0.866547101900567,0.499095301708731,0.));
#29033=DIRECTION('center_axis',(0.,0.,1.));
#29034=DIRECTION('ref_axis',(1.,0.,0.));
#29035=DIRECTION('center_axis',(0.499095301708731,-0.866547101900567,0.));
#29036=DIRECTION('ref_axis',(0.866547101900567,0.499095301708731,0.));
#29037=DIRECTION('',(0.,0.,-1.));
#29038=DIRECTION('',(0.866547101900567,0.499095301708731,0.));
#29039=DIRECTION('center_axis',(0.,0.,1.));
#29040=DIRECTION('ref_axis',(-1.,1.38777878078145E-16,0.));
#29041=DIRECTION('center_axis',(0.,0.,-1.));
#29042=DIRECTION('ref_axis',(1.,0.,0.));
#29043=DIRECTION('center_axis',(0.,0.,-1.));
#29044=DIRECTION('ref_axis',(1.,0.,0.));
#29045=DIRECTION('center_axis',(0.706367935150259,0.707844856018294,0.));
#29046=DIRECTION('ref_axis',(-0.707844856018294,0.706367935150259,0.));
#29047=DIRECTION('',(0.,0.,1.));
#29048=DIRECTION('',(-0.707844856018294,0.706367935150259,0.));
#29049=DIRECTION('',(0.,0.,1.));
#29050=DIRECTION('',(-0.707844856018294,0.706367935150259,0.));
#29051=DIRECTION('center_axis',(0.,0.,1.));
#29052=DIRECTION('ref_axis',(-0.965925826289068,0.258819045102521,0.));
#29053=DIRECTION('center_axis',(0.,0.,1.));
#29054=DIRECTION('ref_axis',(1.,0.,0.));
#29055=DIRECTION('',(0.966195594825111,0.257810148249736,0.));
#29056=DIRECTION('center_axis',(0.257810148249736,-0.966195594825111,0.));
#29057=DIRECTION('ref_axis',(0.966195594825111,0.257810148249736,0.));
#29058=DIRECTION('',(0.,0.,-1.));
#29059=DIRECTION('',(0.966195594825111,0.257810148249736,0.));
#29060=DIRECTION('center_axis',(0.,0.,1.));
#29061=DIRECTION('ref_axis',(-0.965925826289068,0.258819045102521,0.));
#29062=DIRECTION('center_axis',(0.,0.,-1.));
#29063=DIRECTION('ref_axis',(1.,0.,0.));
#29064=DIRECTION('center_axis',(0.865502761139503,0.500904152967308,0.));
#29065=DIRECTION('ref_axis',(-0.500904152967308,0.865502761139503,0.));
#29066=DIRECTION('',(0.,0.,1.));
#29067=DIRECTION('',(-0.500904152967308,0.865502761139503,0.));
#29068=DIRECTION('',(0.,0.,1.));
#29069=DIRECTION('',(-0.500904152967308,0.865502761139503,0.));
#29070=DIRECTION('center_axis',(0.,0.,1.));
#29071=DIRECTION('ref_axis',(-0.866025403784438,0.5,0.));
#29072=DIRECTION('center_axis',(0.,0.,1.));
#29073=DIRECTION('ref_axis',(1.,0.,0.));
#29074=DIRECTION('',(0.999999454676039,-0.00104434076106422,0.));
#29075=DIRECTION('center_axis',(-0.00104434076106422,-0.999999454676039,
0.));
#29076=DIRECTION('ref_axis',(0.999999454676039,-0.00104434076106422,0.));
#29077=DIRECTION('',(0.,0.,-1.));
#29078=DIRECTION('',(0.999999454676039,-0.00104434076106422,0.));
#29079=DIRECTION('center_axis',(0.,0.,1.));
#29080=DIRECTION('ref_axis',(-0.866025403784438,0.5,0.));
#29081=DIRECTION('center_axis',(0.,0.,-1.));
#29082=DIRECTION('ref_axis',(1.,0.,0.));
#29083=DIRECTION('center_axis',(0.96565500426803,0.259827659674852,0.));
#29084=DIRECTION('ref_axis',(-0.259827659674852,0.96565500426803,0.));
#29085=DIRECTION('',(0.,0.,1.));
#29086=DIRECTION('',(-0.259827659674852,0.96565500426803,0.));
#29087=DIRECTION('',(0.,0.,1.));
#29088=DIRECTION('',(-0.259827659674852,0.96565500426803,0.));
#29089=DIRECTION('center_axis',(0.,0.,1.));
#29090=DIRECTION('ref_axis',(-0.707106781186548,0.707106781186548,0.));
#29091=DIRECTION('center_axis',(0.,0.,1.));
#29092=DIRECTION('ref_axis',(1.,0.,0.));
#29093=DIRECTION('',(0.96565500426803,-0.259827659674852,0.));
#29094=DIRECTION('center_axis',(-0.259827659674852,-0.96565500426803,0.));
#29095=DIRECTION('ref_axis',(0.96565500426803,-0.259827659674852,0.));
#29096=DIRECTION('',(0.,0.,-1.));
#29097=DIRECTION('',(0.96565500426803,-0.259827659674852,0.));
#29098=DIRECTION('center_axis',(0.,0.,1.));
#29099=DIRECTION('ref_axis',(-0.707106781186548,0.707106781186548,0.));
#29100=DIRECTION('center_axis',(0.,0.,-1.));
#29101=DIRECTION('ref_axis',(1.,0.,0.));
#29102=DIRECTION('center_axis',(0.999999454676039,0.00104434076106355,0.));
#29103=DIRECTION('ref_axis',(-0.00104434076106355,0.999999454676039,0.));
#29104=DIRECTION('',(0.,0.,1.));
#29105=DIRECTION('',(-0.00104434076106355,0.999999454676039,0.));
#29106=DIRECTION('',(0.,0.,1.));
#29107=DIRECTION('',(-0.00104434076106355,0.999999454676039,0.));
#29108=DIRECTION('center_axis',(0.,0.,1.));
#29109=DIRECTION('ref_axis',(-0.5,0.866025403784439,0.));
#29110=DIRECTION('center_axis',(0.,0.,1.));
#29111=DIRECTION('ref_axis',(1.,0.,0.));
#29112=DIRECTION('',(0.865502761139503,-0.500904152967308,0.));
#29113=DIRECTION('center_axis',(-0.500904152967309,-0.865502761139503,0.));
#29114=DIRECTION('ref_axis',(0.865502761139503,-0.500904152967309,0.));
#29115=DIRECTION('',(0.,0.,-1.));
#29116=DIRECTION('',(0.865502761139503,-0.500904152967308,0.));
#29117=DIRECTION('center_axis',(0.,0.,1.));
#29118=DIRECTION('ref_axis',(-0.5,0.866025403784439,0.));
#29119=DIRECTION('center_axis',(0.,0.,-1.));
#29120=DIRECTION('ref_axis',(1.,0.,0.));
#29121=DIRECTION('center_axis',(0.966195594825111,-0.257810148249736,0.));
#29122=DIRECTION('ref_axis',(0.257810148249736,0.966195594825111,0.));
#29123=DIRECTION('',(0.,0.,1.));
#29124=DIRECTION('',(0.257810148249736,0.966195594825111,0.));
#29125=DIRECTION('',(0.,0.,1.));
#29126=DIRECTION('',(0.257810148249736,0.966195594825111,0.));
#29127=DIRECTION('center_axis',(0.,0.,1.));
#29128=DIRECTION('ref_axis',(-0.258819045102521,0.965925826289068,0.));
#29129=DIRECTION('center_axis',(0.,0.,1.));
#29130=DIRECTION('ref_axis',(1.,0.,0.));
#29131=DIRECTION('',(0.706367935150259,-0.707844856018294,0.));
#29132=DIRECTION('center_axis',(-0.707844856018294,-0.706367935150259,0.));
#29133=DIRECTION('ref_axis',(0.706367935150259,-0.707844856018294,0.));
#29134=DIRECTION('',(0.,0.,-1.));
#29135=DIRECTION('',(0.706367935150259,-0.707844856018294,0.));
#29136=DIRECTION('center_axis',(0.,0.,1.));
#29137=DIRECTION('ref_axis',(-0.258819045102521,0.965925826289068,0.));
#29138=DIRECTION('center_axis',(0.,0.,-1.));
#29139=DIRECTION('ref_axis',(1.,0.,0.));
#29140=DIRECTION('center_axis',(0.866547101900567,-0.499095301708731,0.));
#29141=DIRECTION('ref_axis',(0.499095301708731,0.866547101900567,0.));
#29142=DIRECTION('',(0.,0.,1.));
#29143=DIRECTION('',(0.499095301708731,0.866547101900567,0.));
#29144=DIRECTION('',(0.,0.,1.));
#29145=DIRECTION('',(0.499095301708731,0.866547101900567,0.));
#29146=DIRECTION('center_axis',(0.,0.,1.));
#29147=DIRECTION('ref_axis',(8.32667268468867E-17,1.,0.));
#29148=DIRECTION('center_axis',(0.,0.,1.));
#29149=DIRECTION('ref_axis',(1.,0.,0.));
#29150=DIRECTION('',(0.499095301708731,-0.866547101900567,0.));
#29151=DIRECTION('center_axis',(-0.866547101900567,-0.499095301708731,0.));
#29152=DIRECTION('ref_axis',(0.499095301708731,-0.866547101900567,0.));
#29153=DIRECTION('',(0.,0.,-1.));
#29154=DIRECTION('',(0.499095301708731,-0.866547101900567,0.));
#29155=DIRECTION('center_axis',(0.,0.,1.));
#29156=DIRECTION('ref_axis',(8.32667268468867E-17,1.,0.));
#29157=DIRECTION('center_axis',(0.,0.,-1.));
#29158=DIRECTION('ref_axis',(1.,0.,0.));
#29159=DIRECTION('center_axis',(0.707844856018294,-0.706367935150259,0.));
#29160=DIRECTION('ref_axis',(0.706367935150259,0.707844856018294,0.));
#29161=DIRECTION('',(0.,0.,1.));
#29162=DIRECTION('',(0.706367935150259,0.707844856018294,0.));
#29163=DIRECTION('',(0.,0.,1.));
#29164=DIRECTION('',(0.706367935150259,0.707844856018294,0.));
#29165=DIRECTION('center_axis',(0.,0.,1.));
#29166=DIRECTION('ref_axis',(0.258819045102521,0.965925826289068,0.));
#29167=DIRECTION('center_axis',(0.,0.,1.));
#29168=DIRECTION('ref_axis',(1.,0.,0.));
#29169=DIRECTION('',(0.257810148249736,-0.966195594825111,0.));
#29170=DIRECTION('center_axis',(-0.966195594825111,-0.257810148249736,0.));
#29171=DIRECTION('ref_axis',(0.257810148249736,-0.966195594825111,0.));
#29172=DIRECTION('',(0.,0.,-1.));
#29173=DIRECTION('',(0.257810148249736,-0.966195594825111,0.));
#29174=DIRECTION('center_axis',(0.,0.,1.));
#29175=DIRECTION('ref_axis',(0.258819045102521,0.965925826289068,0.));
#29176=DIRECTION('center_axis',(0.,0.,-1.));
#29177=DIRECTION('ref_axis',(1.,0.,0.));
#29178=DIRECTION('center_axis',(0.500904152967308,-0.865502761139503,0.));
#29179=DIRECTION('ref_axis',(0.865502761139503,0.500904152967308,0.));
#29180=DIRECTION('',(0.,0.,1.));
#29181=DIRECTION('',(0.865502761139503,0.500904152967308,0.));
#29182=DIRECTION('',(0.,0.,1.));
#29183=DIRECTION('',(0.865502761139503,0.500904152967308,0.));
#29184=DIRECTION('center_axis',(0.,0.,1.));
#29185=DIRECTION('ref_axis',(0.5,0.866025403784439,0.));
#29186=DIRECTION('center_axis',(0.,0.,1.));
#29187=DIRECTION('ref_axis',(1.,0.,0.));
#29188=DIRECTION('',(-0.00104434076106397,-0.999999454676039,0.));
#29189=DIRECTION('center_axis',(-0.999999454676039,0.00104434076106394,
0.));
#29190=DIRECTION('ref_axis',(-0.00104434076106394,-0.999999454676039,0.));
#29191=DIRECTION('',(0.,0.,-1.));
#29192=DIRECTION('',(-0.00104434076106397,-0.999999454676039,0.));
#29193=DIRECTION('center_axis',(0.,0.,1.));
#29194=DIRECTION('ref_axis',(0.5,0.866025403784439,0.));
#29195=DIRECTION('center_axis',(0.,0.,-1.));
#29196=DIRECTION('ref_axis',(1.,0.,0.));
#29197=DIRECTION('center_axis',(0.259827659674852,-0.96565500426803,0.));
#29198=DIRECTION('ref_axis',(0.96565500426803,0.259827659674852,0.));
#29199=DIRECTION('',(0.,0.,1.));
#29200=DIRECTION('',(0.96565500426803,0.259827659674852,0.));
#29201=DIRECTION('',(0.,0.,1.));
#29202=DIRECTION('',(0.96565500426803,0.259827659674852,0.));
#29203=DIRECTION('center_axis',(0.,0.,1.));
#29204=DIRECTION('ref_axis',(0.707106781186547,0.707106781186548,0.));
#29205=DIRECTION('center_axis',(0.,0.,1.));
#29206=DIRECTION('ref_axis',(1.,0.,0.));
#29207=DIRECTION('',(-0.259827659674852,-0.96565500426803,0.));
#29208=DIRECTION('center_axis',(-0.96565500426803,0.259827659674852,0.));
#29209=DIRECTION('ref_axis',(-0.259827659674852,-0.96565500426803,0.));
#29210=DIRECTION('',(0.,0.,-1.));
#29211=DIRECTION('',(-0.259827659674852,-0.96565500426803,0.));
#29212=DIRECTION('center_axis',(0.,0.,1.));
#29213=DIRECTION('ref_axis',(0.707106781186547,0.707106781186548,0.));
#29214=DIRECTION('center_axis',(0.,0.,-1.));
#29215=DIRECTION('ref_axis',(1.,0.,0.));
#29216=DIRECTION('center_axis',(0.00104434076106372,-0.999999454676039,
0.));
#29217=DIRECTION('ref_axis',(0.999999454676039,0.00104434076106372,0.));
#29218=DIRECTION('',(0.,0.,1.));
#29219=DIRECTION('',(0.999999454676039,0.00104434076106372,0.));
#29220=DIRECTION('',(0.,0.,1.));
#29221=DIRECTION('',(0.999999454676039,0.00104434076106372,0.));
#29222=DIRECTION('center_axis',(0.,0.,1.));
#29223=DIRECTION('ref_axis',(0.866025403784439,0.5,0.));
#29224=DIRECTION('center_axis',(0.,0.,1.));
#29225=DIRECTION('ref_axis',(1.,0.,0.));
#29226=DIRECTION('',(-0.500904152967308,-0.865502761139503,0.));
#29227=DIRECTION('center_axis',(-0.865502761139503,0.500904152967308,0.));
#29228=DIRECTION('ref_axis',(-0.500904152967308,-0.865502761139503,0.));
#29229=DIRECTION('',(0.,0.,-1.));
#29230=DIRECTION('',(-0.500904152967308,-0.865502761139503,0.));
#29231=DIRECTION('center_axis',(0.,0.,1.));
#29232=DIRECTION('ref_axis',(0.866025403784439,0.5,0.));
#29233=DIRECTION('center_axis',(0.,0.,-1.));
#29234=DIRECTION('ref_axis',(1.,0.,0.));
#29235=DIRECTION('center_axis',(-0.257810148249736,-0.966195594825111,0.));
#29236=DIRECTION('ref_axis',(0.966195594825111,-0.257810148249736,0.));
#29237=DIRECTION('',(0.,0.,1.));
#29238=DIRECTION('',(0.966195594825111,-0.257810148249736,0.));
#29239=DIRECTION('',(0.,0.,1.));
#29240=DIRECTION('',(0.966195594825111,-0.257810148249736,0.));
#29241=DIRECTION('center_axis',(0.,0.,1.));
#29242=DIRECTION('ref_axis',(0.965925826289068,0.258819045102521,0.));
#29243=DIRECTION('center_axis',(0.,0.,1.));
#29244=DIRECTION('ref_axis',(1.,0.,0.));
#29245=DIRECTION('',(-0.707844856018294,-0.706367935150259,0.));
#29246=DIRECTION('center_axis',(-0.706367935150259,0.707844856018294,0.));
#29247=DIRECTION('ref_axis',(-0.707844856018294,-0.706367935150259,0.));
#29248=DIRECTION('',(0.,0.,-1.));
#29249=DIRECTION('',(-0.707844856018294,-0.706367935150259,0.));
#29250=DIRECTION('center_axis',(0.,0.,1.));
#29251=DIRECTION('ref_axis',(0.965925826289068,0.258819045102521,0.));
#29252=DIRECTION('center_axis',(0.,0.,-1.));
#29253=DIRECTION('ref_axis',(1.,0.,0.));
#29254=DIRECTION('center_axis',(-0.499095301708731,-0.866547101900567,0.));
#29255=DIRECTION('ref_axis',(0.866547101900567,-0.499095301708731,0.));
#29256=DIRECTION('',(0.,0.,1.));
#29257=DIRECTION('',(0.866547101900567,-0.499095301708731,0.));
#29258=DIRECTION('',(0.,0.,1.));
#29259=DIRECTION('',(0.866547101900567,-0.499095301708731,0.));
#29260=DIRECTION('center_axis',(0.,0.,1.));
#29261=DIRECTION('ref_axis',(1.,0.,0.));
#29262=DIRECTION('center_axis',(0.,0.,1.));
#29263=DIRECTION('ref_axis',(1.,0.,0.));
#29264=DIRECTION('',(-0.866547101900567,-0.499095301708731,0.));
#29265=DIRECTION('center_axis',(-0.499095301708731,0.866547101900567,0.));
#29266=DIRECTION('ref_axis',(-0.866547101900567,-0.499095301708731,0.));
#29267=DIRECTION('',(0.,0.,-1.));
#29268=DIRECTION('',(-0.866547101900567,-0.499095301708731,0.));
#29269=DIRECTION('center_axis',(0.,0.,1.));
#29270=DIRECTION('ref_axis',(1.,0.,0.));
#29271=DIRECTION('center_axis',(0.,0.,-1.));
#29272=DIRECTION('ref_axis',(1.,0.,0.));
#29273=DIRECTION('center_axis',(0.,0.,-1.));
#29274=DIRECTION('ref_axis',(-1.,0.,0.));
#29275=DIRECTION('center_axis',(0.,0.,1.));
#29276=DIRECTION('ref_axis',(1.,0.,0.));
#29277=DIRECTION('center_axis',(0.,0.,1.));
#29278=DIRECTION('ref_axis',(1.,0.,0.));
#29279=DIRECTION('',(0.707106781186547,8.65956056235493E-17,-0.707106781186548));
#29280=DIRECTION('center_axis',(0.,0.,-1.));
#29281=DIRECTION('ref_axis',(-1.,0.,0.));
#29282=DIRECTION('center_axis',(0.,0.,1.));
#29283=DIRECTION('ref_axis',(1.,0.,0.));
#29284=DIRECTION('center_axis',(0.,0.,1.));
#29285=DIRECTION('ref_axis',(1.,0.,0.));
#29286=DIRECTION('center_axis',(0.,0.,1.));
#29287=DIRECTION('ref_axis',(1.,0.,0.));
#29288=DIRECTION('',(0.707106781186547,8.65956056235493E-17,-0.707106781186548));
#29289=DIRECTION('center_axis',(0.,0.,1.));
#29290=DIRECTION('ref_axis',(1.,0.,0.));
#29291=DIRECTION('center_axis',(0.,0.,1.));
#29292=DIRECTION('ref_axis',(1.,0.,0.));
#29293=DIRECTION('',(0.,0.,-1.));
#29294=DIRECTION('',(0.,0.,-1.));
#29295=DIRECTION('center_axis',(0.,0.,-1.));
#29296=DIRECTION('ref_axis',(1.,0.,0.));
#29297=DIRECTION('center_axis',(0.,0.,1.));
#29298=DIRECTION('ref_axis',(1.,0.,0.));
#29299=DIRECTION('',(-0.707106781186548,-8.65956056235493E-17,-0.707106781186547));
#29300=DIRECTION('center_axis',(0.,0.,1.));
#29301=DIRECTION('ref_axis',(1.,0.,0.));
#36156=CARTESIAN_POINT('',(0.,0.,0.));
#36157=CARTESIAN_POINT('Origin',(0.,0.,-0.56));
#36158=CARTESIAN_POINT('',(-0.195084575036282,1.57151725016375E-5,-0.962013030787577));
#36159=CARTESIAN_POINT('',(-0.195110174310067,3.211721741748E-6,-0.972186969212424));
#36160=CARTESIAN_POINT('',(-0.1954,-2.39295984553393E-17,-0.56));
#36161=CARTESIAN_POINT('',(0.188713086871761,-0.0519137165493658,-1.));
#36162=CARTESIAN_POINT('Ctrl Pts',(-0.195084575036282,1.57151725016375E-5,
-0.962013030787577));
#36163=CARTESIAN_POINT('Ctrl Pts',(-0.195109875732101,0.0316848016664486,
-0.963811747031453));
#36164=CARTESIAN_POINT('Ctrl Pts',(-0.187839688942379,0.0633440313364852,
-0.96561046327533));
#36165=CARTESIAN_POINT('Ctrl Pts',(-0.173214336083063,0.0911354430469698,
-0.967409179519207));
#36166=CARTESIAN_POINT('Ctrl Pts',(-0.143076407955131,0.148404185672271,
-0.97111572809974));
#36167=CARTESIAN_POINT('Ctrl Pts',(-0.0817059931899262,0.189248884082378,
-0.974822276680274));
#36168=CARTESIAN_POINT('Ctrl Pts',(-0.0172563726780756,0.194958105016696,
-0.978528825260807));
#36169=CARTESIAN_POINT('Ctrl Pts',(0.0471932478337753,0.200667325951015,
-0.98223537384134));
#36170=CARTESIAN_POINT('Ctrl Pts',(0.114722074092272,0.171241069409545,
-0.985941922421872));
#36171=CARTESIAN_POINT('Ctrl Pts',(0.154471393616461,0.120160647611379,
-0.989648471002406));
#36172=CARTESIAN_POINT('Ctrl Pts',(0.191474931611372,0.0726087309639927,
-0.993098980668271));
#36173=CARTESIAN_POINT('Ctrl Pts',(0.204404282404944,0.00629095093881454,
-0.996549490334136));
#36174=CARTESIAN_POINT('Ctrl Pts',(0.188715001522267,-0.0519146961985303,
-1.));
#36175=CARTESIAN_POINT('',(-0.1954,-2.39295984553393E-17,-1.));
#36176=CARTESIAN_POINT('Origin',(0.,0.,-1.));
#36177=CARTESIAN_POINT('',(-0.1954,-2.39295984553393E-17,-1.1246));
#36178=CARTESIAN_POINT('',(-0.1954,-2.39295984553393E-17,-0.56));
#36179=CARTESIAN_POINT('Origin',(0.,0.,-1.1246));
#36180=CARTESIAN_POINT('',(0.156132246633334,0.117489921104866,-1.));
#36181=CARTESIAN_POINT('Origin',(0.,0.,-1.));
#36182=CARTESIAN_POINT('Ctrl Pts',(0.156132246633334,0.117489921104866,
-1.));
#36183=CARTESIAN_POINT('Ctrl Pts',(0.117043464717142,0.169434966955124,
-0.996293451419467));
#36184=CARTESIAN_POINT('Ctrl Pts',(0.050333107650634,0.199889556663511,
-0.992586902838933));
#36185=CARTESIAN_POINT('Ctrl Pts',(-0.0141001197016129,0.195197543652393,
-0.9888803542584));
#36186=CARTESIAN_POINT('Ctrl Pts',(-0.0785333470538611,0.190505530641275,
-0.985173805677867));
#36187=CARTESIAN_POINT('Ctrl Pts',(-0.140689444691848,0.15066691491065,
-0.981467257097333));
#36188=CARTESIAN_POINT('Ctrl Pts',(-0.17177246279413,0.0938911568835147,
-0.9777607085168));
#36189=CARTESIAN_POINT('Ctrl Pts',(-0.187352872792911,0.06543222200327,
-0.975902795415341));
#36190=CARTESIAN_POINT('Ctrl Pts',(-0.19512607572876,0.0327177778867662,
-0.974044882313883));
#36191=CARTESIAN_POINT('Ctrl Pts',(-0.195110174310067,3.211721741748E-6,
-0.972186969212424));
#36192=CARTESIAN_POINT('Origin',(0.,0.,-0.56));
#36193=CARTESIAN_POINT('',(-0.195426264375126,-0.000177548476699763,-0.892013030787577));
#36194=CARTESIAN_POINT('',(-0.195457760643607,-0.000174238830481377,-0.902186969212424));
#36195=CARTESIAN_POINT('',(-0.1954,-2.39295984553393E-17,-0.56));
#36196=CARTESIAN_POINT('Ctrl Pts',(-0.195426264375126,-0.000177548476699763,
-0.892013030787577));
#36197=CARTESIAN_POINT('Ctrl Pts',(-0.194957410957457,0.050526042153958,
-0.894905788881586));
#36198=CARTESIAN_POINT('Ctrl Pts',(-0.174765431648993,0.101560768688629,
-0.897798546975596));
#36199=CARTESIAN_POINT('Ctrl Pts',(-0.139284034569977,0.137501909669616,
-0.900691305069606));
#36200=CARTESIAN_POINT('Ctrl Pts',(-0.09382101356905,0.183554009691976,
-0.904397853650139));
#36201=CARTESIAN_POINT('Ctrl Pts',(-0.0232561208383973,0.204825751547922,
-0.908104402230672));
#36202=CARTESIAN_POINT('Ctrl Pts',(0.0400842191953776,0.191572593489572,
-0.911810950811206));
#36203=CARTESIAN_POINT('Ctrl Pts',(0.103424559229153,0.178319435431222,
-0.915517499391739));
#36204=CARTESIAN_POINT('Ctrl Pts',(0.159540346566049,0.130541377458575,
-0.919224047972273));
#36205=CARTESIAN_POINT('Ctrl Pts',(0.182726664407761,0.0701254468485091,
-0.922930596552806));
#36206=CARTESIAN_POINT('Ctrl Pts',(0.205912982249472,0.00970951623844284,
-0.92663714513334));
#36207=CARTESIAN_POINT('Ctrl Pts',(0.196169830595998,-0.063344287009043,
-0.930343693713872));
#36208=CARTESIAN_POINT('Ctrl Pts',(0.157957512983411,-0.115570247816891,
-0.934050242294406));
#36209=CARTESIAN_POINT('Ctrl Pts',(0.119745195370824,-0.167796208624739,
-0.937756790874939));
#36210=CARTESIAN_POINT('Ctrl Pts',(0.0530637117991234,-0.199194326992949,
-0.941463339455473));
#36211=CARTESIAN_POINT('Ctrl Pts',(-0.0115345925566828,-0.195381124160082,
-0.945169888036006));
#36212=CARTESIAN_POINT('Ctrl Pts',(-0.0761328969124891,-0.191567921327216,
-0.94887643661654));
#36213=CARTESIAN_POINT('Ctrl Pts',(-0.138648022052401,-0.152543397293271,
-0.952582985197073));
#36214=CARTESIAN_POINT('Ctrl Pts',(-0.170452863877028,-0.0961847418560505,
-0.956289533777606));
#36215=CARTESIAN_POINT('Ctrl Pts',(-0.18682343190734,-0.0671758504419905,
-0.958197366114263));
#36216=CARTESIAN_POINT('Ctrl Pts',(-0.195057739516345,-0.0335745231384176,
-0.96010519845092));
#36217=CARTESIAN_POINT('Ctrl Pts',(-0.195084575036282,1.57151725016375E-5,
-0.962013030787577));
#36218=CARTESIAN_POINT('Ctrl Pts',(-0.195110174310067,3.211721741748E-6,
-0.972186969212424));
#36219=CARTESIAN_POINT('Ctrl Pts',(-0.195094352296248,-0.0325479919097508,
-0.970338333733349));
#36220=CARTESIAN_POINT('Ctrl Pts',(-0.187367022603641,-0.0650993163738915,
-0.968489698254274));
#36221=CARTESIAN_POINT('Ctrl Pts',(-0.171946018101075,-0.0934588054226745,
-0.9666410627752));
#36222=CARTESIAN_POINT('Ctrl Pts',(-0.14102661673916,-0.150320109378084,
-0.962934514194666));
#36223=CARTESIAN_POINT('Ctrl Pts',(-0.0791778754487514,-0.190329816965257,
-0.959227965614133));
#36224=CARTESIAN_POINT('Ctrl Pts',(-0.0146572328544997,-0.195170717064559,
-0.9555214170336));
#36225=CARTESIAN_POINT('Ctrl Pts',(0.049863409739752,-0.200011617163861,
-0.951814868453067));
#36226=CARTESIAN_POINT('Ctrl Pts',(0.117055953637847,-0.169683709775292,
-0.948108319872533));
#36227=CARTESIAN_POINT('Ctrl Pts',(0.156100413855611,-0.11807427426149,
-0.944401771292));
#36228=CARTESIAN_POINT('Ctrl Pts',(0.195144874073376,-0.0664648387476884,
-0.940695222711466));
#36229=CARTESIAN_POINT('Ctrl Pts',(0.206041250610809,0.00642612489134668,
-0.936988674130933));
#36230=CARTESIAN_POINT('Ctrl Pts',(0.183818523921417,0.0672043779064316,
-0.933282125550399));
#36231=CARTESIAN_POINT('Ctrl Pts',(0.161595797232025,0.127982630921516,
-0.929575576969866));
#36232=CARTESIAN_POINT('Ctrl Pts',(0.106253967315808,0.176648173312651,
-0.925869028389332));
#36233=CARTESIAN_POINT('Ctrl Pts',(0.0431341771381354,0.190909062306829,
-0.922162479808799));
#36234=CARTESIAN_POINT('Ctrl Pts',(-0.0199856130395371,0.205169951301007,
-0.918455931228266));
#36235=CARTESIAN_POINT('Ctrl Pts',(-0.0908833634786639,0.185026186898227,
-0.914749382647733));
#36236=CARTESIAN_POINT('Ctrl Pts',(-0.137075323273913,0.139704726559351,
-0.9110428340672));
#36237=CARTESIAN_POINT('Ctrl Pts',(-0.173863343578693,0.103609986033525,
-0.908090879115608));
#36238=CARTESIAN_POINT('Ctrl Pts',(-0.194981009616801,0.0515455718136115,
-0.905138924164016));
#36239=CARTESIAN_POINT('Ctrl Pts',(-0.195457760643607,-0.000174238830481377,
-0.902186969212424));
#36240=CARTESIAN_POINT('Origin',(0.,0.,-0.56));
#36241=CARTESIAN_POINT('',(-0.195673584877587,8.71017904331833E-5,-0.822013030787576));
#36242=CARTESIAN_POINT('',(-0.195653454845991,0.000103118138519916,-0.832186969212424));
#36243=CARTESIAN_POINT('',(-0.1954,-2.39295984553393E-17,-0.56));
#36244=CARTESIAN_POINT('Ctrl Pts',(-0.195673584877587,8.71017904331833E-5,
-0.822013030787576));
#36245=CARTESIAN_POINT('Ctrl Pts',(-0.195700838558998,0.00498315558351734,
-0.822293282151186));
#36246=CARTESIAN_POINT('Ctrl Pts',(-0.195533017114237,0.00987731022659859,
-0.822573533514795));
#36247=CARTESIAN_POINT('Ctrl Pts',(-0.195164122119264,0.0147562617970676,
-0.822853784878405));
#36248=CARTESIAN_POINT('Ctrl Pts',(-0.190285190568779,0.0792843011439578,
-0.826560333458938));
#36249=CARTESIAN_POINT('Ctrl Pts',(-0.150234112753965,0.141152991744968,
-0.830266882039473));
#36250=CARTESIAN_POINT('Ctrl Pts',(-0.0933581745971609,0.172020446737902,
-0.833973430620006));
#36251=CARTESIAN_POINT('Ctrl Pts',(-0.0364822364403571,0.202887901730835,
-0.83767997920054));
#36252=CARTESIAN_POINT('Ctrl Pts',(0.0372185620584375,0.202754121115692,
-0.841386527781072));
#36253=CARTESIAN_POINT('Ctrl Pts',(0.0939820585112729,0.171680389196942,
-0.845093076361605));
#36254=CARTESIAN_POINT('Ctrl Pts',(0.150745554964109,0.140606657278192,
-0.848799624942138));
#36255=CARTESIAN_POINT('Ctrl Pts',(0.190571749370985,0.0785929740558366,
-0.852506173522672));
#36256=CARTESIAN_POINT('Ctrl Pts',(0.195216398313037,0.0140476477414276,
-0.856212722103206));
#36257=CARTESIAN_POINT('Ctrl Pts',(0.199861047255089,-0.0504976785729813,
-0.859919270683739));
#36258=CARTESIAN_POINT('Ctrl Pts',(0.169324150732317,-0.117574647979443,
-0.863625819264272));
#36259=CARTESIAN_POINT('Ctrl Pts',(0.117594518889292,-0.156455475350819,
-0.867332367844806));
#36260=CARTESIAN_POINT('Ctrl Pts',(0.0658648870462679,-0.195336302722196,
-0.871038916425339));
#36261=CARTESIAN_POINT('Ctrl Pts',(-0.00705748011700841,-0.206020988058488,
-0.874745465005873));
#36262=CARTESIAN_POINT('Ctrl Pts',(-0.0677669148374835,-0.183614902949219,
-0.878452013586406));
#36263=CARTESIAN_POINT('Ctrl Pts',(-0.128476349557959,-0.161208817839951,
-0.882158562166939));
#36264=CARTESIAN_POINT('Ctrl Pts',(-0.176972851835633,-0.105711962285121,
-0.885865110747472));
#36265=CARTESIAN_POINT('Ctrl Pts',(-0.19104052833887,-0.0425473054133194,
-0.889571659328006));
#36266=CARTESIAN_POINT('Ctrl Pts',(-0.194129154066305,-0.0286792025866717,
-0.890385449814529));
#36267=CARTESIAN_POINT('Ctrl Pts',(-0.195558162182849,-0.0144414787283386,
-0.891199240301053));
#36268=CARTESIAN_POINT('Ctrl Pts',(-0.195426264375126,-0.000177548476699763,
-0.892013030787577));
#36269=CARTESIAN_POINT('Ctrl Pts',(-0.195457760643607,-0.000174238830481377,
-0.902186969212424));
#36270=CARTESIAN_POINT('Ctrl Pts',(-0.195579630148162,-0.0133951179570571,
-0.901432375583482));
#36271=CARTESIAN_POINT('Ctrl Pts',(-0.194352736283242,-0.0265934792504939,
-0.900677781954541));
#36272=CARTESIAN_POINT('Ctrl Pts',(-0.191694052762859,-0.0394968154586175,
-0.899923188325599));
#36273=CARTESIAN_POINT('Ctrl Pts',(-0.178634653305186,-0.102877740862738,
-0.896216639745066));
#36274=CARTESIAN_POINT('Ctrl Pts',(-0.13102968523847,-0.159140435396007,
-0.892510091164533));
#36275=CARTESIAN_POINT('Ctrl Pts',(-0.0706852958104853,-0.182511338506239,
-0.888803542584));
#36276=CARTESIAN_POINT('Ctrl Pts',(-0.0103409063825001,-0.20588224161647,
-0.885096994003466));
#36277=CARTESIAN_POINT('Ctrl Pts',(0.0627429044067541,-0.196361353303663,
-0.881390445422932));
#36278=CARTESIAN_POINT('Ctrl Pts',(0.115085809889437,-0.15831004487468,
-0.877683896842399));
#36279=CARTESIAN_POINT('Ctrl Pts',(0.167428715372121,-0.120258736445697,
-0.873977348261865));
#36280=CARTESIAN_POINT('Ctrl Pts',(0.199030715548233,-0.0536770079005367,
-0.870270799681332));
#36281=CARTESIAN_POINT('Ctrl Pts',(0.195415447752892,0.0109341586965677,
-0.866564251100799));
#36282=CARTESIAN_POINT('Ctrl Pts',(0.191800179957551,0.0755453252936721,
-0.862857702520266));
#36283=CARTESIAN_POINT('Ctrl Pts',(0.152967644190756,0.138185929942721,
-0.859151153939732));
#36284=CARTESIAN_POINT('Ctrl Pts',(0.0967066977677326,0.170160507747372,
-0.855444605359199));
#36285=CARTESIAN_POINT('Ctrl Pts',(0.0404457513447093,0.202135085552022,
-0.851738056778666));
#36286=CARTESIAN_POINT('Ctrl Pts',(-0.0332436057345425,0.203443636512275,
-0.848031508198133));
#36287=CARTESIAN_POINT('Ctrl Pts',(-0.0906043506555229,0.173486699003936,
-0.844324959617599));
#36288=CARTESIAN_POINT('Ctrl Pts',(-0.147965095576503,0.143529761495597,
-0.840618411037066));
#36289=CARTESIAN_POINT('Ctrl Pts',(-0.188997228339212,0.0823073355186673,
-0.836911862456532));
#36290=CARTESIAN_POINT('Ctrl Pts',(-0.194904097710687,0.0178652652725652,
-0.833205313875999));
#36291=CARTESIAN_POINT('Ctrl Pts',(-0.195445052795288,0.0119636169764026,
-0.832865865654807));
#36292=CARTESIAN_POINT('Ctrl Pts',(-0.195691411591684,0.00603496545921146,
-0.832526417433615));
#36293=CARTESIAN_POINT('Ctrl Pts',(-0.195653454845991,0.000103118138519916,
-0.832186969212424));
#36294=CARTESIAN_POINT('Origin',(0.,0.,-0.56));
#36295=CARTESIAN_POINT('',(-0.195164384848501,0.000125606292110517,-0.752013030787577));
#36296=CARTESIAN_POINT('',(-0.195145082735841,0.000112707534856574,-0.762186969212424));
#36297=CARTESIAN_POINT('',(-0.1954,-2.39295984553393E-17,-0.56));
#36298=CARTESIAN_POINT('Ctrl Pts',(-0.195164384848501,0.000125606292110517,
-0.752013030787577));
#36299=CARTESIAN_POINT('Ctrl Pts',(-0.195306581362487,0.0242959090730286,
-0.753387324001319));
#36300=CARTESIAN_POINT('Ctrl Pts',(-0.191149350064068,0.0484190333677505,
-0.754761617215062));
#36301=CARTESIAN_POINT('Ctrl Pts',(-0.182471342534317,0.0707883572077772,
-0.756135910428805));
#36302=CARTESIAN_POINT('Ctrl Pts',(-0.15906625243447,0.131119722230631,
-0.759842459009338));
#36303=CARTESIAN_POINT('Ctrl Pts',(-0.102776483832904,0.178693728526212,
-0.763549007589872));
#36304=CARTESIAN_POINT('Ctrl Pts',(-0.0393882338062579,0.191716846977238,
-0.767255556170405));
#36305=CARTESIAN_POINT('Ctrl Pts',(0.0240000162203877,0.204739965428263,
-0.770962104750938));
#36306=CARTESIAN_POINT('Ctrl Pts',(0.0944867476721127,0.183212196034733,
-0.774668653331471));
#36307=CARTESIAN_POINT('Ctrl Pts',(0.139782170988598,0.136995354217524,
-0.778375201912005));
#36308=CARTESIAN_POINT('Ctrl Pts',(0.185077594305083,0.0907785124003164,
-0.782081750492538));
#36309=CARTESIAN_POINT('Ctrl Pts',(0.205181709486329,0.0198725981594313,
-0.785788299073072));
#36310=CARTESIAN_POINT('Ctrl Pts',(0.190884874109968,-0.0432405727492172,
-0.789494847653606));
#36311=CARTESIAN_POINT('Ctrl Pts',(0.176588038733607,-0.106353743657866,
-0.793201396234139));
#36312=CARTESIAN_POINT('Ctrl Pts',(0.127890252799637,-0.161674171234278,
-0.796907944814671));
#36313=CARTESIAN_POINT('Ctrl Pts',(0.06709984464803,-0.183859710843263,
-0.800614493395204));
#36314=CARTESIAN_POINT('Ctrl Pts',(0.00630943649642266,-0.206045250452247,
-0.804321041975738));
#36315=CARTESIAN_POINT('Ctrl Pts',(-0.0665735938728228,-0.195095902093804,
-0.808027590556272));
#36316=CARTESIAN_POINT('Ctrl Pts',(-0.118161716414366,-0.156027533868197,
-0.811734139136806));
#36317=CARTESIAN_POINT('Ctrl Pts',(-0.165849271791013,-0.119913116799936,
-0.81516043635373));
#36318=CARTESIAN_POINT('Ctrl Pts',(-0.195340386810088,-0.0597710743450758,
-0.818586733570653));
#36319=CARTESIAN_POINT('Ctrl Pts',(-0.195673584877587,8.71017904331833E-5,
-0.822013030787576));
#36320=CARTESIAN_POINT('Ctrl Pts',(-0.195653454845991,0.000103118138519916,
-0.832186969212424));
#36321=CARTESIAN_POINT('Ctrl Pts',(-0.19527694919923,-0.0587368580291033,
-0.828819868853082));
#36322=CARTESIAN_POINT('Ctrl Pts',(-0.166925729961675,-0.117891279502673,
-0.825452768493741));
#36323=CARTESIAN_POINT('Ctrl Pts',(-0.120633753452604,-0.154124226937434,
-0.822085668134399));
#36324=CARTESIAN_POINT('Ctrl Pts',(-0.0696749338428048,-0.194009934386057,
-0.818379119553866));
#36325=CARTESIAN_POINT('Ctrl Pts',(0.00302431135703297,-0.206119634768027,
-0.814672570973332));
#36326=CARTESIAN_POINT('Ctrl Pts',(0.0641606288751104,-0.184905903107813,
-0.810966022392799));
#36327=CARTESIAN_POINT('Ctrl Pts',(0.125296946393188,-0.163692171447599,
-0.807259473812265));
#36328=CARTESIAN_POINT('Ctrl Pts',(0.174870336229504,-0.109155007745201,
-0.803552925231732));
#36329=CARTESIAN_POINT('Ctrl Pts',(0.19017136590337,-0.0462777468575458,
-0.799846376651198));
#36330=CARTESIAN_POINT('Ctrl Pts',(0.205472395577236,0.0165995140301098,
-0.796139828070665));
#36331=CARTESIAN_POINT('Ctrl Pts',(0.186501065088651,0.0878168721030228,
-0.792433279490132));
#36332=CARTESIAN_POINT('Ctrl Pts',(0.141948087059648,0.134749840714092,
-0.788726730909599));
#36333=CARTESIAN_POINT('Ctrl Pts',(0.0973951090306438,0.181682809325161,
-0.785020182329065));
#36334=CARTESIAN_POINT('Ctrl Pts',(0.0272604834612217,0.204331388474385,
-0.781313633748532));
#36335=CARTESIAN_POINT('Ctrl Pts',(-0.0363272967462341,0.192320322314275,
-0.777607085167998));
#36336=CARTESIAN_POINT('Ctrl Pts',(-0.0999150769536897,0.180309256154165,
-0.773900536587465));
#36337=CARTESIAN_POINT('Ctrl Pts',(-0.156956011799179,0.133638544684719,
-0.770193988006932));
#36338=CARTESIAN_POINT('Ctrl Pts',(-0.181319798015859,0.0736879202010541,
-0.766487439426399));
#36339=CARTESIAN_POINT('Ctrl Pts',(-0.190742376698605,0.050502300722489,
-0.765053949355074));
#36340=CARTESIAN_POINT('Ctrl Pts',(-0.195277372458642,0.025330379538085,
-0.763620459283749));
#36341=CARTESIAN_POINT('Ctrl Pts',(-0.195145082735841,0.000112707534856574,
-0.762186969212424));
#36342=CARTESIAN_POINT('Origin',(0.,0.,-0.56));
#36343=CARTESIAN_POINT('',(-0.195216518518634,-0.000150737487880678,-0.682013030787577));
#36344=CARTESIAN_POINT('',(-0.195242183955992,-0.000159443835737465,-0.692186969212424));
#36345=CARTESIAN_POINT('',(-0.1954,-2.39295984553393E-17,-0.56));
#36346=CARTESIAN_POINT('Ctrl Pts',(-0.195216518518634,-0.000150737487880678,
-0.682013030787577));
#36347=CARTESIAN_POINT('Ctrl Pts',(-0.194904732781107,0.0432318296131434,
-0.684481365851453));
#36348=CARTESIAN_POINT('Ctrl Pts',(-0.180636578142957,0.0868005498567561,
-0.686949700915328));
#36349=CARTESIAN_POINT('Ctrl Pts',(-0.154055925496942,0.120720976604095,
-0.689418035979204));
#36350=CARTESIAN_POINT('Ctrl Pts',(-0.114141376707916,0.171657217575372,
-0.693124584559738));
#36351=CARTESIAN_POINT('Ctrl Pts',(-0.0464631280272487,0.200837327099895,
-0.696831133140271));
#36352=CARTESIAN_POINT('Ctrl Pts',(0.0179755900401639,0.1948939725487,-0.700537681720805));
#36353=CARTESIAN_POINT('Ctrl Pts',(0.0824143081075773,0.188950617997505,
-0.704244230301338));
#36354=CARTESIAN_POINT('Ctrl Pts',(0.143613495561735,0.14788379937059,-0.707950778881872));
#36355=CARTESIAN_POINT('Ctrl Pts',(0.173537963060344,0.0905061199632647,
-0.711657327462405));
#36356=CARTESIAN_POINT('Ctrl Pts',(0.203462430558953,0.0331284405559403,
-0.715363876042938));
#36357=CARTESIAN_POINT('Ctrl Pts',(0.202112178102014,-0.0405600996317941,
-0.719070424623471));
#36358=CARTESIAN_POINT('Ctrl Pts',(0.17010575285896,-0.0968029711114258,
-0.722776973204005));
#36359=CARTESIAN_POINT('Ctrl Pts',(0.138099327615907,-0.153045842591058,
-0.726483521784538));
#36360=CARTESIAN_POINT('Ctrl Pts',(0.0754367295867393,-0.191843045362587,
-0.730190070365071));
#36361=CARTESIAN_POINT('Ctrl Pts',(0.0108235326741567,-0.195421681278553,
-0.733896618945605));
#36362=CARTESIAN_POINT('Ctrl Pts',(-0.0537896642384258,-0.199000317194519,
-0.737603167526138));
#36363=CARTESIAN_POINT('Ctrl Pts',(-0.120353460034423,-0.167360386254922,
-0.741309716106672));
#36364=CARTESIAN_POINT('Ctrl Pts',(-0.158375152133358,-0.114996058910061,
-0.745016264687205));
#36365=CARTESIAN_POINT('Ctrl Pts',(-0.182299375309043,-0.082047082031722,
-0.747348520053995));
#36366=CARTESIAN_POINT('Ctrl Pts',(-0.194923069109207,-0.0408928007072448,
-0.749680775420786));
#36367=CARTESIAN_POINT('Ctrl Pts',(-0.195164384848501,0.000125606292110517,
-0.752013030787577));
#36368=CARTESIAN_POINT('Ctrl Pts',(-0.195145082735841,0.000112707534856574,
-0.762186969212424));
#36369=CARTESIAN_POINT('Ctrl Pts',(-0.194935313386121,-0.0398744853142615,
-0.759913910703216));
#36370=CARTESIAN_POINT('Ctrl Pts',(-0.182990189434058,-0.079976713355511,
-0.757640852194007));
#36371=CARTESIAN_POINT('Ctrl Pts',(-0.160188039888451,-0.11245697275395,
-0.755367793684799));
#36372=CARTESIAN_POINT('Ctrl Pts',(-0.12300585795649,-0.165420703727406,
-0.751661245104265));
#36373=CARTESIAN_POINT('Ctrl Pts',(-0.0569548565046961,-0.198117628176434,
-0.747954696523731));
#36374=CARTESIAN_POINT('Ctrl Pts',(0.00770717133859991,-0.195569369605572,
-0.744248147943198));
#36375=CARTESIAN_POINT('Ctrl Pts',(0.0723691991818959,-0.19302111103471,
-0.740541599362665));
#36376=CARTESIAN_POINT('Ctrl Pts',(0.135642253416694,-0.155227669443958,
-0.736835050782132));
#36377=CARTESIAN_POINT('Ctrl Pts',(0.168541111895386,-0.0995021226113438,
-0.733128502201599));
#36378=CARTESIAN_POINT('Ctrl Pts',(0.201439970374078,-0.0437765757787303,
-0.729421953621065));
#36379=CARTESIAN_POINT('Ctrl Pts',(0.203964633096664,0.0298810762957444,
-0.725715405040532));
#36380=CARTESIAN_POINT('Ctrl Pts',(0.174958558506099,0.0877284539034402,
-0.722008856459998));
#36381=CARTESIAN_POINT('Ctrl Pts',(0.145952483915533,0.145575831511137,
-0.718302307879465));
#36382=CARTESIAN_POINT('Ctrl Pts',(0.0854156720118136,0.187612934652054,
-0.714595759298931));
#36383=CARTESIAN_POINT('Ctrl Pts',(0.0210798796572213,0.194582675199021,
-0.710889210718398));
#36384=CARTESIAN_POINT('Ctrl Pts',(-0.0432559126973706,0.201552415745988,
-0.707182662137865));
#36385=CARTESIAN_POINT('Ctrl Pts',(-0.111390685502836,0.173454793699006,
-0.703476113557332));
#36386=CARTESIAN_POINT('Ctrl Pts',(-0.152112075758141,0.123161256980201,
-0.699769564976798));
#36387=CARTESIAN_POINT('Ctrl Pts',(-0.179880392163595,0.0888655997837939,
-0.69724203305534));
#36388=CARTESIAN_POINT('Ctrl Pts',(-0.194901457733376,0.0442488196347122,
-0.694714501133882));
#36389=CARTESIAN_POINT('Ctrl Pts',(-0.195242183955992,-0.000159443835737465,
-0.692186969212424));
#36390=CARTESIAN_POINT('Origin',(0.,0.,-0.56));
#36391=CARTESIAN_POINT('',(-0.195707701541145,-4.64929517365598E-5,-0.612013030787577));
#36392=CARTESIAN_POINT('',(-0.195716357106892,-2.76508156398553E-5,-0.622186969212424));
#36393=CARTESIAN_POINT('',(-0.1954,-2.39295984553393E-17,-0.56));
#36394=CARTESIAN_POINT('Ctrl Pts',(-0.195707701541145,-4.64929517365598E-5,
-0.612013030787577));
#36395=CARTESIAN_POINT('Ctrl Pts',(-0.195508230414245,0.0621601619704314,
-0.615575407701586));
#36396=CARTESIAN_POINT('Ctrl Pts',(-0.163290136797982,0.124544569513887,
-0.619137784615595));
#36397=CARTESIAN_POINT('Ctrl Pts',(-0.112366285628439,0.160251677767253,
-0.622700161529604));
#36398=CARTESIAN_POINT('Ctrl Pts',(-0.0593815137123928,0.197403875472946,
-0.626406710110138));
#36399=CARTESIAN_POINT('Ctrl Pts',(0.0138537212886752,0.205675785227547,
-0.630113258690671));
#36400=CARTESIAN_POINT('Ctrl Pts',(0.0737905478189984,0.181278066587556,
-0.633819807271204));
#36401=CARTESIAN_POINT('Ctrl Pts',(0.133727374349322,0.156880347947566,
-0.637526355851737));
#36402=CARTESIAN_POINT('Ctrl Pts',(0.180365792408901,0.0998130009129835,
-0.641232904432271));
#36403=CARTESIAN_POINT('Ctrl Pts',(0.192340863426324,0.0362184294191327,
-0.644939453012805));
#36404=CARTESIAN_POINT('Ctrl Pts',(0.204315934443746,-0.0273761420747171,
-0.648646001593338));
#36405=CARTESIAN_POINT('Ctrl Pts',(0.181627658419013,-0.097497938027835,
-0.652352550173871));
#36406=CARTESIAN_POINT('Ctrl Pts',(0.134669475861856,-0.142024345251873,
-0.656059098754404));
#36407=CARTESIAN_POINT('Ctrl Pts',(0.0877112933047003,-0.186550752475911,
-0.659765647334937));
#36408=CARTESIAN_POINT('Ctrl Pts',(0.0164832042151199,-0.20548177097087,
-0.663472195915471));
#36409=CARTESIAN_POINT('Ctrl Pts',(-0.0463853881973819,-0.190145150174586,
-0.667178744496004));
#36410=CARTESIAN_POINT('Ctrl Pts',(-0.109253980609885,-0.174808529378301,
-0.670885293076538));
#36411=CARTESIAN_POINT('Ctrl Pts',(-0.163763076345309,-0.125204269290772,
-0.674591841657071));
#36412=CARTESIAN_POINT('Ctrl Pts',(-0.18494219976433,-0.0640559530379924,
-0.678298390237604));
#36413=CARTESIAN_POINT('Ctrl Pts',(-0.192017320005872,-0.0436286822063926,
-0.679536603754262));
#36414=CARTESIAN_POINT('Ctrl Pts',(-0.195372922452669,-0.0219131318070045,
-0.680774817270919));
#36415=CARTESIAN_POINT('Ctrl Pts',(-0.195216518518634,-0.000150737487880678,
-0.682013030787577));
#36416=CARTESIAN_POINT('Ctrl Pts',(-0.195242183955992,-0.000159443835737465,
-0.692186969212424));
#36417=CARTESIAN_POINT('Ctrl Pts',(-0.195401122361176,-0.0208745461803437,
-0.691007952553348));
#36418=CARTESIAN_POINT('Ctrl Pts',(-0.192365709442112,-0.0415442765813754,
-0.689828935894273));
#36419=CARTESIAN_POINT('Ctrl Pts',(-0.185939734982374,-0.0610998671791814,
-0.688649919235198));
#36420=CARTESIAN_POINT('Ctrl Pts',(-0.165737996246156,-0.122578003229134,
-0.684943370654664));
#36421=CARTESIAN_POINT('Ctrl Pts',(-0.112026511068576,-0.173044823938413,
-0.681236822074131));
#36422=CARTESIAN_POINT('Ctrl Pts',(-0.0494103717638331,-0.189381609392125,
-0.677530273493598));
#36423=CARTESIAN_POINT('Ctrl Pts',(0.01320576754091,-0.205718394845837,
-0.673823724913065));
#36424=CARTESIAN_POINT('Ctrl Pts',(0.0847265609728156,-0.187925145043982,
-0.670117176332531));
#36425=CARTESIAN_POINT('Ctrl Pts',(0.132388518224354,-0.144152901656579,
-0.666410627751998));
#36426=CARTESIAN_POINT('Ctrl Pts',(0.180050475475893,-0.100380658269176,
-0.662704079171464));
#36427=CARTESIAN_POINT('Ctrl Pts',(0.203853596547065,-0.0306294212962258,
-0.658997530590931));
#36428=CARTESIAN_POINT('Ctrl Pts',(0.192893733296786,0.0331479481837195,
-0.655290982010398));
#36429=CARTESIAN_POINT('Ctrl Pts',(0.181933870046508,0.0969253176636644,
-0.651584433429865));
#36430=CARTESIAN_POINT('Ctrl Pts',(0.136211022474779,0.154728819650604,
-0.647877884849331));
#36431=CARTESIAN_POINT('Ctrl Pts',(0.0766707086837813,0.180078819531201,
-0.644171336268798));
#36432=CARTESIAN_POINT('Ctrl Pts',(0.017130394892783,0.205428819411797,
-0.640464787688264));
#36433=CARTESIAN_POINT('Ctrl Pts',(-0.0562273851174842,0.198325317186049,
-0.636758239107731));
#36434=CARTESIAN_POINT('Ctrl Pts',(-0.10979762224029,0.162022408833456,
-0.633051690527198));
#36435=CARTESIAN_POINT('Ctrl Pts',(-0.16213973013031,0.126551766033109,
-0.629430116755607));
#36436=CARTESIAN_POINT('Ctrl Pts',(-0.195591177290711,0.0632051975665141,
-0.625808542984015));
#36437=CARTESIAN_POINT('Ctrl Pts',(-0.195716357106892,-2.76508156398553E-5,
-0.622186969212424));
#36438=CARTESIAN_POINT('Origin',(0.,0.,-0.56));
#36439=CARTESIAN_POINT('',(-0.195354221420379,0.000178407506690854,-0.542013030787577));
#36440=CARTESIAN_POINT('',(-0.195323759319157,0.000175885597776871,-0.552186969212423));
#36441=CARTESIAN_POINT('',(-0.1954,-2.39295984553393E-17,-0.56));
#36442=CARTESIAN_POINT('Ctrl Pts',(-0.195354221420379,0.000178407506690854,
-0.542013030787577));
#36443=CARTESIAN_POINT('Ctrl Pts',(-0.195503876356803,0.0168432028806296,
-0.542962900971186));
#36444=CARTESIAN_POINT('Ctrl Pts',(-0.193549298846388,0.033473417735259,
-0.543912771154795));
#36445=CARTESIAN_POINT('Ctrl Pts',(-0.189353619137088,0.0495175654979228,
-0.544862641338404));
#36446=CARTESIAN_POINT('Ctrl Pts',(-0.172981391711447,0.112124450250982,
-0.548569189918937));
#36447=CARTESIAN_POINT('Ctrl Pts',(-0.122484173387406,0.165807362599245,
-0.55227573849947));
#36448=CARTESIAN_POINT('Ctrl Pts',(-0.0609946091473485,0.185974299375253,
-0.555982287080004));
#36449=CARTESIAN_POINT('Ctrl Pts',(0.00049495509270836,0.206141236151261,
-0.559688835660537));
#36450=CARTESIAN_POINT('Ctrl Pts',(0.0729768652487818,0.192792197355014,
-0.56339538424107));
#36451=CARTESIAN_POINT('Ctrl Pts',(0.123247345926238,0.15204234309985,-0.567101932821604));
#36452=CARTESIAN_POINT('Ctrl Pts',(0.173517826603694,0.111292488844685,
-0.570808481402137));
#36453=CARTESIAN_POINT('Ctrl Pts',(0.201576877802532,0.043141819130602,
-0.57451502998267));
#36454=CARTESIAN_POINT('Ctrl Pts',(0.194570720810425,-0.0211900206811239,
-0.578221578563204));
#36455=CARTESIAN_POINT('Ctrl Pts',(0.187564563818317,-0.0855218604928506,
-0.581928127143737));
#36456=CARTESIAN_POINT('Ctrl Pts',(0.145493198635262,-0.14603487040222,
-0.58563467572427));
#36457=CARTESIAN_POINT('Ctrl Pts',(0.0876294087333888,-0.175008197231417,
-0.589341224304804));
#36458=CARTESIAN_POINT('Ctrl Pts',(0.0297656188315169,-0.203981524060614,
-0.593047772885337));
#36459=CARTESIAN_POINT('Ctrl Pts',(-0.043890595789172,-0.201415167809638,
-0.596754321465871));
#36460=CARTESIAN_POINT('Ctrl Pts',(-0.099597513898962,-0.168484769633043,
-0.600460870046404));
#36461=CARTESIAN_POINT('Ctrl Pts',(-0.155304432008752,-0.135554371456448,
-0.604167418626937));
#36462=CARTESIAN_POINT('Ctrl Pts',(-0.193062053607643,-0.0722599313542328,
-0.607873967207471));
#36463=CARTESIAN_POINT('Ctrl Pts',(-0.195573709991577,-0.00759646847473161,
-0.611580515788004));
#36464=CARTESIAN_POINT('Ctrl Pts',(-0.195671404566122,-0.00508128784131614,
-0.611724687454528));
#36465=CARTESIAN_POINT('Ctrl Pts',(-0.195715774264914,-0.00256403596459507,
-0.611868859121052));
#36466=CARTESIAN_POINT('Ctrl Pts',(-0.195707701541145,-4.64929517365598E-5,
-0.612013030787577));
#36467=CARTESIAN_POINT('Ctrl Pts',(-0.195716357106892,-2.76508156398553E-5,
-0.622186969212424));
#36468=CARTESIAN_POINT('Ctrl Pts',(-0.195719294263949,-0.00151131497631132,
-0.622101994403482));
#36469=CARTESIAN_POINT('Ctrl Pts',(-0.195703884111172,-0.00299491652998268,
-0.62201701959454));
#36470=CARTESIAN_POINT('Ctrl Pts',(-0.195669940176563,-0.00447809392031211,
-0.621932044785597));
#36471=CARTESIAN_POINT('Ctrl Pts',(-0.194189326754688,-0.0691733738420494,
-0.618225496205064));
#36472=CARTESIAN_POINT('Ctrl Pts',(-0.157445405675594,-0.133061619206086,
-0.614518947624531));
#36473=CARTESIAN_POINT('Ctrl Pts',(-0.102270472059719,-0.166875790210921,
-0.610812399043998));
#36474=CARTESIAN_POINT('Ctrl Pts',(-0.0470955384438438,-0.200689961215756,
-0.607105850463464));
#36475=CARTESIAN_POINT('Ctrl Pts',(0.0265104077088127,-0.20443005786139,
-0.603399301882931));
#36476=CARTESIAN_POINT('Ctrl Pts',(0.084828673023672,-0.176382751557177,
-0.599692753302397));
#36477=CARTESIAN_POINT('Ctrl Pts',(0.143146938338532,-0.148335445252965,
-0.595986204721864));
#36478=CARTESIAN_POINT('Ctrl Pts',(0.186177522815594,-0.0885007359989063,
-0.592279656141331));
#36479=CARTESIAN_POINT('Ctrl Pts',(0.194208227107422,-0.0242887491986593,
-0.588573107560798));
#36480=CARTESIAN_POINT('Ctrl Pts',(0.202238931399251,0.0399232376015871,
-0.584866558980264));
#36481=CARTESIAN_POINT('Ctrl Pts',(0.175269755505846,0.108512501948022,
-0.58116001039973));
#36482=CARTESIAN_POINT('Ctrl Pts',(0.125655209083708,0.15005847941376,-0.577453461819197));
#36483=CARTESIAN_POINT('Ctrl Pts',(0.0760406626615685,0.191604456879499,
-0.573746913238664));
#36484=CARTESIAN_POINT('Ctrl Pts',(0.00378074571069509,0.20610714746454,
-0.570040364658131));
#36485=CARTESIAN_POINT('Ctrl Pts',(-0.0580224608868743,0.186922906157784,
-0.566333816077598));
#36486=CARTESIAN_POINT('Ctrl Pts',(-0.119825667484444,0.167738664851027,
-0.562627267497064));
#36487=CARTESIAN_POINT('Ctrl Pts',(-0.171172163728709,0.114867491652473,
-0.55892071891653));
#36488=CARTESIAN_POINT('Ctrl Pts',(-0.188540252620716,0.0525295341266019,
-0.555214170335997));
#36489=CARTESIAN_POINT('Ctrl Pts',(-0.193268523595349,0.0355587115438646,
-0.554205103294806));
#36490=CARTESIAN_POINT('Ctrl Pts',(-0.195478516591736,0.0178862670678721,
-0.553196036253614));
#36491=CARTESIAN_POINT('Ctrl Pts',(-0.195323759319157,0.000175885597776871,
-0.552186969212423));
#36492=CARTESIAN_POINT('Origin',(0.,0.,-0.56));
#36493=CARTESIAN_POINT('',(-0.195092696479446,-5.43760739497856E-5,-0.472013030787576));
#36494=CARTESIAN_POINT('',(-0.195102639049386,-7.04728118876389E-5,-0.482186969212424));
#36495=CARTESIAN_POINT('',(-0.1954,-2.39295984553393E-17,-0.56));
#36496=CARTESIAN_POINT('Ctrl Pts',(-0.195092696479446,-5.43760739497856E-5,
-0.472013030787576));
#36497=CARTESIAN_POINT('Ctrl Pts',(-0.195003108324315,0.0359258718284784,
-0.474056942821319));
#36498=CARTESIAN_POINT('Ctrl Pts',(-0.185481340256412,0.0719502167704471,
-0.476100854855061));
#36499=CARTESIAN_POINT('Ctrl Pts',(-0.166817881086069,0.102364920373673,
-0.478144766888803));
#36500=CARTESIAN_POINT('Ctrl Pts',(-0.132972482187457,0.157520707221052,
-0.481851315469337));
#36501=CARTESIAN_POINT('Ctrl Pts',(-0.0690634452147766,0.194228460215231,
-0.48555786404987));
#36502=CARTESIAN_POINT('Ctrl Pts',(-0.00436733455159703,0.195672452741996,
-0.489264412630403));
#36503=CARTESIAN_POINT('Ctrl Pts',(0.0603287761115817,0.197116445268761,
-0.492970961210936));
#36504=CARTESIAN_POINT('Ctrl Pts',(0.125811960465259,0.163296677328114,
-0.49667750979147));
#36505=CARTESIAN_POINT('Ctrl Pts',(0.162084541285929,0.109705897057926,
-0.500384058372003));
#36506=CARTESIAN_POINT('Ctrl Pts',(0.198357122106599,0.0561151167877383,
-0.504090606952537));
#36507=CARTESIAN_POINT('Ctrl Pts',(0.205419099394263,-0.0172466758119902,
-0.50779715553307));
#36508=CARTESIAN_POINT('Ctrl Pts',(0.180035399636139,-0.0767726334771048,
-0.511503704113603));
#36509=CARTESIAN_POINT('Ctrl Pts',(0.154651699878015,-0.136298591142221,
-0.515210252694137));
#36510=CARTESIAN_POINT('Ctrl Pts',(0.0968223230741041,-0.181988713872723,
-0.51891680127467));
#36511=CARTESIAN_POINT('Ctrl Pts',(0.0330387570242473,-0.192912474732577,
-0.522623349855203));
#36512=CARTESIAN_POINT('Ctrl Pts',(-0.0307448090256087,-0.20383623559243,
-0.526329898435737));
#36513=CARTESIAN_POINT('Ctrl Pts',(-0.100482564321409,-0.179993634581636,
-0.53003644701627));
#36514=CARTESIAN_POINT('Ctrl Pts',(-0.144227823705689,-0.132306905497313,
-0.533742995596803));
#36515=CARTESIAN_POINT('Ctrl Pts',(-0.176762568331955,-0.0968407641449097,
-0.536499673993728));
#36516=CARTESIAN_POINT('Ctrl Pts',(-0.194919898354602,-0.0481855502101019,
-0.539256352390652));
#36517=CARTESIAN_POINT('Ctrl Pts',(-0.195354221420379,0.000178407506690854,
-0.542013030787577));
#36518=CARTESIAN_POINT('Ctrl Pts',(-0.195323759319157,0.000175885597776871,
-0.552186969212423));
#36519=CARTESIAN_POINT('Ctrl Pts',(-0.194910055502839,-0.0471682700629787,
-0.549489487673081));
#36520=CARTESIAN_POINT('Ctrl Pts',(-0.177597305086522,-0.0947835321655527,
-0.546792006133739));
#36521=CARTESIAN_POINT('Ctrl Pts',(-0.146318441124281,-0.129991125084758,
-0.544094524594397));
#36522=CARTESIAN_POINT('Ctrl Pts',(-0.10333885919609,-0.17836908491706,
-0.540387976013864));
#36523=CARTESIAN_POINT('Ctrl Pts',(-0.0339900137999589,-0.203320262728478,
-0.53668142743333));
#36524=CARTESIAN_POINT('Ctrl Pts',(0.0299595685248398,-0.193414588559514,
-0.532974878852797));
#36525=CARTESIAN_POINT('Ctrl Pts',(0.0939091508496379,-0.183508914390551,
-0.529268330272263));
#36526=CARTESIAN_POINT('Ctrl Pts',(0.152459470103104,-0.138746388241206,
-0.52556178169173));
#36527=CARTESIAN_POINT('Ctrl Pts',(0.178788776615697,-0.0796326074551339,
-0.521855233111197));
#36528=CARTESIAN_POINT('Ctrl Pts',(0.205118083128289,-0.0205188266690613,
-0.518148684530664));
#36529=CARTESIAN_POINT('Ctrl Pts',(0.199226376900009,0.0529462087537386,
-0.51444213595013));
#36530=CARTESIAN_POINT('Ctrl Pts',(0.163812633301037,0.107108356279148,
-0.510735587369597));
#36531=CARTESIAN_POINT('Ctrl Pts',(0.128398889702065,0.161270503804557,
-0.507029038789064));
#36532=CARTESIAN_POINT('Ctrl Pts',(0.0634631087324024,0.196129763432576,
-0.50332249020853));
#36533=CARTESIAN_POINT('Ctrl Pts',(-0.00124779645749392,0.195717198574478,
-0.499615941627997));
#36534=CARTESIAN_POINT('Ctrl Pts',(-0.0659587016473898,0.19530463371638,
-0.495909393047463));
#36535=CARTESIAN_POINT('Ctrl Pts',(-0.13044473105752,0.159620244372166,
-0.49220284446693));
#36536=CARTESIAN_POINT('Ctrl Pts',(-0.16516500156249,0.105010956917379,
-0.488496295886397));
#36537=CARTESIAN_POINT('Ctrl Pts',(-0.184865406945462,0.0740254523436011,
-0.486393186995072));
#36538=CARTESIAN_POINT('Ctrl Pts',(-0.194982821215997,0.0369471372026458,
-0.484290078103748));
#36539=CARTESIAN_POINT('Ctrl Pts',(-0.195102639049386,-7.04728118876389E-5,
-0.482186969212424));
#36540=CARTESIAN_POINT('Origin',(0.,0.,-0.56));
#36541=CARTESIAN_POINT('',(-0.195553853432401,-0.000152262014626814,-0.402013030787576));
#36542=CARTESIAN_POINT('',(-0.195582229504364,-0.000141746448570984,-0.412186969212424));
#36543=CARTESIAN_POINT('',(-0.1954,-2.39295984553393E-17,-0.56));
#36544=CARTESIAN_POINT('Ctrl Pts',(-0.195553853432401,-0.000152262014626814,
-0.402013030787576));
#36545=CARTESIAN_POINT('Ctrl Pts',(-0.195082861820371,0.054756524969974,
-0.405150984671452));
#36546=CARTESIAN_POINT('Ctrl Pts',(-0.170885527056883,0.110028797080402,
-0.408288938555327));
#36547=CARTESIAN_POINT('Ctrl Pts',(-0.129908286827409,0.146392005883943,
-0.411426892439203));
#36548=CARTESIAN_POINT('Ctrl Pts',(-0.0815060039298814,0.189344198606403,
-0.415133441019736));
#36549=CARTESIAN_POINT('Ctrl Pts',(-0.00969186798292979,0.2059138701436,
-0.418839989600269));
#36550=CARTESIAN_POINT('Ctrl Pts',(0.0526362512551988,0.188510496861456,
-0.422546538180803));
#36551=CARTESIAN_POINT('Ctrl Pts',(0.114964370493328,0.171107123579313,
-0.426253086761336));
#36552=CARTESIAN_POINT('Ctrl Pts',(0.167806473022633,0.119730705477828,
-0.42995963534187));
#36553=CARTESIAN_POINT('Ctrl Pts',(0.18695572847696,0.0579166466812693,
-0.433666183922403));
#36554=CARTESIAN_POINT('Ctrl Pts',(0.206104983931288,-0.00389741211528853,
-0.437372732502936));
#36555=CARTESIAN_POINT('Ctrl Pts',(0.191561392310639,-0.0761491116069204,
-0.441079281083469));
#36556=CARTESIAN_POINT('Ctrl Pts',(0.149987335284637,-0.125740135308376,
-0.444785829664003));
#36557=CARTESIAN_POINT('Ctrl Pts',(0.108413278258634,-0.175331159009831,
-0.448492378244536));
#36558=CARTESIAN_POINT('Ctrl Pts',(0.0398087558272775,-0.20226150692111,
-0.45219892682507));
#36559=CARTESIAN_POINT('Ctrl Pts',(-0.0243986778933489,-0.194194456383829,
-0.455905475405603));
#36560=CARTESIAN_POINT('Ctrl Pts',(-0.0886061116139757,-0.186127405846548,
-0.459612023986136));
#36561=CARTESIAN_POINT('Ctrl Pts',(-0.148416456623872,-0.143062956860706,
-0.46331857256667));
#36562=CARTESIAN_POINT('Ctrl Pts',(-0.176430748716548,-0.084728822017495,
-0.467025121147203));
#36563=CARTESIAN_POINT('Ctrl Pts',(-0.18899704451809,-0.0585620357449116,
-0.468687757693994));
#36564=CARTESIAN_POINT('Ctrl Pts',(-0.195165572678823,-0.0293227957209801,
-0.470350394240785));
#36565=CARTESIAN_POINT('Ctrl Pts',(-0.195092696479446,-5.43760739497856E-5,
-0.472013030787576));
#36566=CARTESIAN_POINT('Ctrl Pts',(-0.195102639049386,-7.04728118876389E-5,
-0.482186969212424));
#36567=CARTESIAN_POINT('Ctrl Pts',(-0.195193989844546,-0.0282932174076707,
-0.480583529523215));
#36568=CARTESIAN_POINT('Ctrl Pts',(-0.189473986501732,-0.0564806756233877,
-0.478980089834006));
#36569=CARTESIAN_POINT('Ctrl Pts',(-0.177758887424744,-0.0819057797433008,
-0.477376650144797));
#36570=CARTESIAN_POINT('Ctrl Pts',(-0.150677991182218,-0.140679043383832,
-0.473670101564263));
#36571=CARTESIAN_POINT('Ctrl Pts',(-0.091561687097356,-0.184691385099535,
-0.46996355298373));
#36572=CARTESIAN_POINT('Ctrl Pts',(-0.0274910010256872,-0.193780865093658,
-0.466257004403196));
#36573=CARTESIAN_POINT('Ctrl Pts',(0.0365796850459811,-0.202870345087781,
-0.462550455822663));
#36574=CARTESIAN_POINT('Ctrl Pts',(0.105604753104456,-0.177036963360327,
-0.45884390724213));
#36575=CARTESIAN_POINT('Ctrl Pts',(0.14796399817062,-0.128114925200796,
-0.455137358661597));
#36576=CARTESIAN_POINT('Ctrl Pts',(0.190323243236784,-0.0791928870412662,
-0.451430810081063));
#36577=CARTESIAN_POINT('Ctrl Pts',(0.206016665310636,-0.00718219244966056,
-0.44772426150053));
#36578=CARTESIAN_POINT('Ctrl Pts',(0.187855148368726,0.0549292458095403,
-0.444017712919996));
#36579=CARTESIAN_POINT('Ctrl Pts',(0.169693631426815,0.117040684068742,
-0.440311164339463));
#36580=CARTESIAN_POINT('Ctrl Pts',(0.117677175469141,0.169252865995539,
-0.43660461575893));
#36581=CARTESIAN_POINT('Ctrl Pts',(0.0556343843049091,0.187647526220983,
-0.432898067178396));
#36582=CARTESIAN_POINT('Ctrl Pts',(-0.00640840685932162,0.206042186446427,
-0.429191518597863));
#36583=CARTESIAN_POINT('Ctrl Pts',(-0.0784775332301094,0.19061932497052,
-0.42548497001733));
#36584=CARTESIAN_POINT('Ctrl Pts',(-0.127558314596203,0.148444114707243,
-0.421778421436796));
#36585=CARTESIAN_POINT('Ctrl Pts',(-0.169893833240166,0.112065121734498,
-0.418581270695339));
#36586=CARTESIAN_POINT('Ctrl Pts',(-0.195125475882863,0.0557817443309313,
-0.415384119953881));
#36587=CARTESIAN_POINT('Ctrl Pts',(-0.195582229504364,-0.000141746448570984,
-0.412186969212424));
#36588=CARTESIAN_POINT('Origin',(0.,0.,-0.56));
#36589=CARTESIAN_POINT('',(-0.195574688910705,0.000144757554679794,-0.332013030787576));
#36590=CARTESIAN_POINT('',(-0.195545913560384,0.000154829267465116,-0.342186969212424));
#36591=CARTESIAN_POINT('',(-0.1954,-2.39295984553393E-17,-0.56));
#36592=CARTESIAN_POINT('Ctrl Pts',(-0.195574688910705,0.000144757554679794,
-0.332013030787576));
#36593=CARTESIAN_POINT('Ctrl Pts',(-0.195650878894854,0.00933662874909953,
-0.332538477941052));
#36594=CARTESIAN_POINT('Ctrl Pts',(-0.195058964365449,0.0185186393964773,
-0.333063925094527));
#36595=CARTESIAN_POINT('Ctrl Pts',(-0.19376528178542,0.0276006874476484,
-0.333589372248002));
#36596=CARTESIAN_POINT('Ctrl Pts',(-0.184639535649099,0.0916662211359821,
-0.337295920828535));
#36597=CARTESIAN_POINT('Ctrl Pts',(-0.140593736189925,0.150757605336143,
-0.341002469409069));
#36598=CARTESIAN_POINT('Ctrl Pts',(-0.0818051501088732,0.177805229925724,
-0.344709017989602));
#36599=CARTESIAN_POINT('Ctrl Pts',(-0.0230165640278225,0.204852854515306,
-0.348415566570136));
#36600=CARTESIAN_POINT('Ctrl Pts',(0.0505148086751044,0.199856719494309,
-0.352122115150669));
#36601=CARTESIAN_POINT('Ctrl Pts',(0.105104436528749,0.165105541382207,
-0.355828663731202));
#36602=CARTESIAN_POINT('Ctrl Pts',(0.159694064382394,0.130354363270105,
-0.359535212311736));
#36603=CARTESIAN_POINT('Ctrl Pts',(0.195341947386756,0.0658481420668959,
-0.363241760892269));
#36604=CARTESIAN_POINT('Ctrl Pts',(0.195717882626462,0.00113701070568482,
-0.366948309472803));
#36605=CARTESIAN_POINT('Ctrl Pts',(0.196093817866168,-0.063574120655523,
-0.370654858053336));
#36606=CARTESIAN_POINT('Ctrl Pts',(0.161197805341222,-0.128490162174734,
-0.374361406633869));
#36607=CARTESIAN_POINT('Ctrl Pts',(0.107015618047075,-0.163873243292415,
-0.378067955214402));
#36608=CARTESIAN_POINT('Ctrl Pts',(0.0528334307529256,-0.199256324410097,
-0.381774503794935));
#36609=CARTESIAN_POINT('Ctrl Pts',(-0.0206349313104262,-0.205106445126249,
-0.385481052375469));
#36610=CARTESIAN_POINT('Ctrl Pts',(-0.0797338016833294,-0.178743680286252,
-0.389187600956003));
#36611=CARTESIAN_POINT('Ctrl Pts',(-0.138832672056233,-0.152380915446255,
-0.392894149536536));
#36612=CARTESIAN_POINT('Ctrl Pts',(-0.183562050738688,-0.093805265050108,
-0.396600698117069));
#36613=CARTESIAN_POINT('Ctrl Pts',(-0.193431525155864,-0.0298500828981727,
-0.400307246697602));
#36614=CARTESIAN_POINT('Ctrl Pts',(-0.194945529543094,-0.0200391829179675,
-0.40087584139426));
#36615=CARTESIAN_POINT('Ctrl Pts',(-0.195639196730193,-0.0101016896463702,
-0.401444436090918));
#36616=CARTESIAN_POINT('Ctrl Pts',(-0.195553853432401,-0.000152262014626814,
-0.402013030787576));
#36617=CARTESIAN_POINT('Ctrl Pts',(-0.195582229504364,-0.000141746448570984,
-0.412186969212424));
#36618=CARTESIAN_POINT('Ctrl Pts',(-0.195655003460488,-0.00905196296956772,
-0.411677571373348));
#36619=CARTESIAN_POINT('Ctrl Pts',(-0.195098851215254,-0.0179530435413701,
-0.411168173534272));
#36620=CARTESIAN_POINT('Ctrl Pts',(-0.193882746133758,-0.0267630260896144,
-0.410658775695196));
#36621=CARTESIAN_POINT('Ctrl Pts',(-0.185033959943818,-0.0908673975725523,
-0.406952227114663));
#36622=CARTESIAN_POINT('Ctrl Pts',(-0.141243951202538,-0.150148581487782,
-0.403245678534129));
#36623=CARTESIAN_POINT('Ctrl Pts',(-0.0825728095466741,-0.177450020956349,
-0.399539129953596));
#36624=CARTESIAN_POINT('Ctrl Pts',(-0.0239016678908108,-0.204751460424916,
-0.395832581373063));
#36625=CARTESIAN_POINT('Ctrl Pts',(0.0496506066796362,-0.200073155446821,
-0.392126032792529));
#36626=CARTESIAN_POINT('Ctrl Pts',(0.104389907602852,-0.165558225420882,
-0.388419484211996));
#36627=CARTESIAN_POINT('Ctrl Pts',(0.159129208526068,-0.131043295394943,
-0.384712935631463));
#36628=CARTESIAN_POINT('Ctrl Pts',(0.195055535802052,-0.0666917403211604,
-0.381006387050929));
#36629=CARTESIAN_POINT('Ctrl Pts',(0.195711131915094,-0.00198284097962335,
-0.377299838470396));
#36630=CARTESIAN_POINT('Ctrl Pts',(0.196366728028137,0.0627260583619147,
-0.373593289889863));
#36631=CARTESIAN_POINT('Ctrl Pts',(0.161751592978236,0.127792301971207,
-0.36988674130933));
#36632=CARTESIAN_POINT('Ctrl Pts',(0.107722830516848,0.163409212100406,
-0.366180192728796));
#36633=CARTESIAN_POINT('Ctrl Pts',(0.0536940680554607,0.199026122229604,
-0.362473644148263));
#36634=CARTESIAN_POINT('Ctrl Pts',(-0.0197483218174141,0.20519369887871,
-0.358767095567729));
#36635=CARTESIAN_POINT('Ctrl Pts',(-0.0789605704353628,0.179086591151826,
-0.355060546987196));
#36636=CARTESIAN_POINT('Ctrl Pts',(-0.138172819053312,0.152979483424941,
-0.351353998406662));
#36637=CARTESIAN_POINT('Ctrl Pts',(-0.183154926416334,0.0945976913220663,
-0.347647449826129));
#36638=CARTESIAN_POINT('Ctrl Pts',(-0.193300705595433,0.0306857626616098,
-0.343940901245596));
#36639=CARTESIAN_POINT('Ctrl Pts',(-0.1949010270011,0.0206047599404502,
-0.343356257234539));
#36640=CARTESIAN_POINT('Ctrl Pts',(-0.19563463405017,0.0103861695630058,
-0.342771613223481));
#36641=CARTESIAN_POINT('Ctrl Pts',(-0.195545913560384,0.000154829267465116,
-0.342186969212424));
#36642=CARTESIAN_POINT('Origin',(0.,0.,-0.56));
#36643=CARTESIAN_POINT('',(-0.195099694633333,6.61648413741723E-5,-0.262013030787576));
#36644=CARTESIAN_POINT('',(-0.195090438596196,4.99224700532782E-5,-0.272186969212423));
#36645=CARTESIAN_POINT('',(-0.1954,-2.39295984553393E-17,-0.56));
#36646=CARTESIAN_POINT('Ctrl Pts',(-0.195099694633333,6.61648413741722E-5,
-0.262013030787576));
#36647=CARTESIAN_POINT('Ctrl Pts',(-0.195186244887412,0.0285724785253478,
-0.263632519791185));
#36648=CARTESIAN_POINT('Ctrl Pts',(-0.189346489992417,0.057045028877643,
-0.265252008794793));
#36649=CARTESIAN_POINT('Ctrl Pts',(-0.17740326045936,0.0826732456169493,
-0.266871497798402));
#36650=CARTESIAN_POINT('Ctrl Pts',(-0.150068613311955,0.141328926615721,
-0.270578046378935));
#36651=CARTESIAN_POINT('Ctrl Pts',(-0.0907626488691269,0.185085374337137,
-0.274284594959468));
#36652=CARTESIAN_POINT('Ctrl Pts',(-0.0266532758367687,0.19389787328715,
-0.277991143540002));
#36653=CARTESIAN_POINT('Ctrl Pts',(0.0374560971955886,0.202710372237162,
-0.281697692120535));
#36654=CARTESIAN_POINT('Ctrl Pts',(0.106368878817475,0.176578922415771,
-0.285404240701069));
#36655=CARTESIAN_POINT('Ctrl Pts',(0.148516302139648,0.127474273373296,
-0.289110789281602));
#36656=CARTESIAN_POINT('Ctrl Pts',(0.190663725461821,0.0783696243308199,
-0.292817337862135));
#36657=CARTESIAN_POINT('Ctrl Pts',(0.20604579048428,0.00629177606725653,
-0.296523886442669));
#36658=CARTESIAN_POINT('Ctrl Pts',(0.187616013061667,-0.0557405957499364,
-0.300230435023202));
#36659=CARTESIAN_POINT('Ctrl Pts',(0.169186235639053,-0.11777296756713,
-0.303936983603735));
#36660=CARTESIAN_POINT('Ctrl Pts',(0.116944615771367,-0.169759862937953,
-0.307643532184269));
#36661=CARTESIAN_POINT('Ctrl Pts',(0.0548229042621313,-0.187886219670852,
-0.311350080764802));
#36662=CARTESIAN_POINT('Ctrl Pts',(-0.00729880724710397,-0.20601257640375,
-0.315056629345336));
#36663=CARTESIAN_POINT('Ctrl Pts',(-0.0793006103978895,-0.190278394498723,
-0.318763177925869));
#36664=CARTESIAN_POINT('Ctrl Pts',(-0.128198665566548,-0.147891461957956,
-0.322469726506402));
#36665=CARTESIAN_POINT('Ctrl Pts',(-0.170164842374355,-0.111513379042165,
-0.32565082793346));
#36666=CARTESIAN_POINT('Ctrl Pts',(-0.195113428314472,-0.0555036066633279,
-0.328831929360518));
#36667=CARTESIAN_POINT('Ctrl Pts',(-0.195574688910705,0.000144757554679794,
-0.332013030787576));
#36668=CARTESIAN_POINT('Ctrl Pts',(-0.195545913560384,0.000154829267465116,
-0.342186969212424));
#36669=CARTESIAN_POINT('Ctrl Pts',(-0.195072160477773,-0.0544788750319072,
-0.339065064642948));
#36670=CARTESIAN_POINT('Ctrl Pts',(-0.171150663017774,-0.109476128897877,
-0.335943160073472));
#36671=CARTESIAN_POINT('Ctrl Pts',(-0.13053973515857,-0.14582920269464,
-0.332821255503996));
#36672=CARTESIAN_POINT('Ctrl Pts',(-0.0823235345474341,-0.188990174172393,
-0.329114706923462));
#36673=CARTESIAN_POINT('Ctrl Pts',(-0.0105816823299884,-0.205870051909861,
-0.325408158342929));
#36674=CARTESIAN_POINT('Ctrl Pts',(0.0518210647242702,-0.188736207614769,
-0.321701609762396));
#36675=CARTESIAN_POINT('Ctrl Pts',(0.11422381177853,-0.171602363319677,
-0.317995061181862));
#36676=CARTESIAN_POINT('Ctrl Pts',(0.167287453669601,-0.120454796992023,
-0.314288512601329));
#36677=CARTESIAN_POINT('Ctrl Pts',(0.186703673424414,-0.0587240763527305,
-0.310581964020795));
#36678=CARTESIAN_POINT('Ctrl Pts',(0.206119893179227,0.00300664428656105,
-0.306875415440262));
#36679=CARTESIAN_POINT('Ctrl Pts',(0.191888690797781,0.0753205192374923,
-0.303168866859729));
#36680=CARTESIAN_POINT('Ctrl Pts',(0.150529343245733,0.125090749601239,
-0.299462318279196));
#36681=CARTESIAN_POINT('Ctrl Pts',(0.109169995693685,0.174860979964985,
-0.295755769698662));
#36682=CARTESIAN_POINT('Ctrl Pts',(0.0406825029710331,0.202087565741548,
-0.292049221118129));
#36683=CARTESIAN_POINT('Ctrl Pts',(-0.0235591918084649,0.19429807846698,
-0.288342672537595));
#36684=CARTESIAN_POINT('Ctrl Pts',(-0.0878008865879639,0.186508591192413,
-0.284636123957062));
#36685=CARTESIAN_POINT('Ctrl Pts',(-0.147796783424309,0.143703030866715,
-0.280929575376528));
#36686=CARTESIAN_POINT('Ctrl Pts',(-0.176062917307789,0.0854905138682907,
-0.277223026795995));
#36687=CARTESIAN_POINT('Ctrl Pts',(-0.188864573152777,0.0591262218304634,
-0.275544340934805));
#36688=CARTESIAN_POINT('Ctrl Pts',(-0.195157947941312,0.029601716953994,
-0.273865655073614));
#36689=CARTESIAN_POINT('Ctrl Pts',(-0.195090438596196,4.99224700532782E-5,
-0.272186969212423));
#36690=CARTESIAN_POINT('Origin',(0.,0.,-0.56));
#36691=CARTESIAN_POINT('',(-0.195331947549774,-0.000176736735444216,-0.192013030787576));
#36692=CARTESIAN_POINT('',(-0.195362592747278,-0.00017879229733782,-0.202186969212423));
#36693=CARTESIAN_POINT('',(-0.1954,-2.39295984553393E-17,-0.56));
#36694=CARTESIAN_POINT('Ctrl Pts',(-0.195331947549774,-0.000176736735444216,
-0.192013030787576));
#36695=CARTESIAN_POINT('Ctrl Pts',(-0.194912364267956,0.0474440407802741,
-0.194726561641318));
#36696=CARTESIAN_POINT('Ctrl Pts',(-0.177373029739348,0.0953415099082568,
-0.19744009249506));
#36697=CARTESIAN_POINT('Ctrl Pts',(-0.14575529320444,0.130622265819019,
-0.200153623348801));
#36698=CARTESIAN_POINT('Ctrl Pts',(-0.102567033040916,0.178814028798557,
-0.203860171929335));
#36699=CARTESIAN_POINT('Ctrl Pts',(-0.0331110015127663,0.203465269351282,
-0.207566720509868));
#36700=CARTESIAN_POINT('Ctrl Pts',(0.0307951764230636,0.193283314489515,
-0.211273269090402));
#36701=CARTESIAN_POINT('Ctrl Pts',(0.0947013543588918,0.183101359627749,
-0.214979817670935));
#36702=CARTESIAN_POINT('Ctrl Pts',(0.153057678702401,0.138086209351492,
-0.218686366251468));
#36703=CARTESIAN_POINT('Ctrl Pts',(0.179131266631905,0.0788591893060497,
-0.222392914832002));
#36704=CARTESIAN_POINT('Ctrl Pts',(0.205204854561408,0.0196321692606077,
-0.226099463412535));
#36705=CARTESIAN_POINT('Ctrl Pts',(0.198995706076907,-0.0538067205540178,
-0.229806011993068));
#36706=CARTESIAN_POINT('Ctrl Pts',(0.163348216926586,-0.107815315807003,
-0.233512560573602));
#36707=CARTESIAN_POINT('Ctrl Pts',(0.127700727776265,-0.161823911059988,
-0.237219109154135));
#36708=CARTESIAN_POINT('Ctrl Pts',(0.0626148979601237,-0.196402211751331,
-0.240925657734668));
#36709=CARTESIAN_POINT('Ctrl Pts',(-0.00209362285706425,-0.19570998734557,
-0.244632206315201));
#36710=CARTESIAN_POINT('Ctrl Pts',(-0.0668021436742531,-0.195017762939809,
-0.248338754895735));
#36711=CARTESIAN_POINT('Ctrl Pts',(-0.13113335549249,-0.159055013436942,
-0.252045303476268));
#36712=CARTESIAN_POINT('Ctrl Pts',(-0.165617296475617,-0.104296181547444,
-0.255751852056802));
#36713=CARTESIAN_POINT('Ctrl Pts',(-0.185034292561122,-0.0734629300648085,
-0.257838911633726));
#36714=CARTESIAN_POINT('Ctrl Pts',(-0.194988156033035,-0.0366703457767274,
-0.259925971210651));
#36715=CARTESIAN_POINT('Ctrl Pts',(-0.195099694633333,6.61648413741722E-5,
-0.262013030787576));
#36716=CARTESIAN_POINT('Ctrl Pts',(-0.195090438596196,4.99224700532782E-5,
-0.272186969212423));
#36717=CARTESIAN_POINT('Ctrl Pts',(-0.195008886897137,-0.0356488248114389,
-0.270159106493081));
#36718=CARTESIAN_POINT('Ctrl Pts',(-0.185645032604243,-0.0713873952352632,
-0.268131243773738));
#36719=CARTESIAN_POINT('Ctrl Pts',(-0.167258709593931,-0.101643016872502,
-0.266103381054395));
#36720=CARTESIAN_POINT('Ctrl Pts',(-0.133651997065978,-0.156944556943723,
-0.262396832473862));
#36721=CARTESIAN_POINT('Ctrl Pts',(-0.069902201079457,-0.193928163415013,
-0.258690283893329));
#36722=CARTESIAN_POINT('Ctrl Pts',(-0.0052129381638058,-0.195651741864263,
-0.254983735312795));
#36723=CARTESIAN_POINT('Ctrl Pts',(0.0594763247518444,-0.197375320313514,
-0.251277186732262));
#36724=CARTESIAN_POINT('Ctrl Pts',(0.125105054596624,-0.163838870740725,
-0.247570638151728));
#36725=CARTESIAN_POINT('Ctrl Pts',(0.161608900190277,-0.110405353957066,
-0.243864089571195));
#36726=CARTESIAN_POINT('Ctrl Pts',(0.19811274578393,-0.0569718371734073,
-0.240157540990662));
#36727=CARTESIAN_POINT('Ctrl Pts',(0.205491707126456,0.016358746821123,
-0.236450992410128));
#36728=CARTESIAN_POINT('Ctrl Pts',(0.180365501023706,0.0759938475038011,
-0.232744443829595));
#36729=CARTESIAN_POINT('Ctrl Pts',(0.155239294920955,0.135628948186481,
-0.229037895249062));
#36730=CARTESIAN_POINT('Ctrl Pts',(0.0976079213729281,0.181568565557309,
-0.225331346668528));
#36731=CARTESIAN_POINT('Ctrl Pts',(0.0338721636032817,0.192767879526438,
-0.221624798087995));
#36732=CARTESIAN_POINT('Ctrl Pts',(-0.0298635941663648,0.203967193495566,
-0.217918249507461));
#36733=CARTESIAN_POINT('Ctrl Pts',(-0.0997037361576298,0.180426204062994,
-0.214211700926928));
#36734=CARTESIAN_POINT('Ctrl Pts',(-0.143654674518915,0.132928978123408,
-0.210505152346395));
#36735=CARTESIAN_POINT('Ctrl Pts',(-0.176532696237839,0.0973981138402943,
-0.207732424635071));
#36736=CARTESIAN_POINT('Ctrl Pts',(-0.194923208118132,0.0484614215119332,
-0.204959696923747));
#36737=CARTESIAN_POINT('Ctrl Pts',(-0.195362592747278,-0.00017879229733782,
-0.202186969212423));
#36738=CARTESIAN_POINT('Origin',(0.,0.,-0.56));
#36739=CARTESIAN_POINT('',(-0.195714505993407,3.28936632279161E-5,-0.122013030787576));
#36740=CARTESIAN_POINT('',(-0.195704662017859,5.15171773276178E-5,-0.132186969212423));
#36741=CARTESIAN_POINT('',(-0.1954,-2.39295984553393E-17,-0.56));
#36742=CARTESIAN_POINT('Ctrl Pts',(-0.195714505993407,3.28936632279162E-5,
-0.122013030787576));
#36743=CARTESIAN_POINT('Ctrl Pts',(-0.195718608760281,0.00179682927824294,
-0.122114054910918));
#36744=CARTESIAN_POINT('Ctrl Pts',(-0.195696828975953,0.00356066088435405,
-0.122215079034259));
#36745=CARTESIAN_POINT('Ctrl Pts',(-0.195648855912775,0.00532377956943465,
-0.122316103157601));
#36746=CARTESIAN_POINT('Ctrl Pts',(-0.193888736811089,0.0700121415501511,
-0.126022651738134));
#36747=CARTESIAN_POINT('Ctrl Pts',(-0.156868879881412,0.133740814262008,
-0.129729200318667));
#36748=CARTESIAN_POINT('Ctrl Pts',(-0.101548282882389,0.167316176473068,
-0.133435748899201));
#36749=CARTESIAN_POINT('Ctrl Pts',(-0.0462276858833664,0.200891538684129,
-0.137142297479734));
#36750=CARTESIAN_POINT('Ctrl Pts',(0.0273936511850024,0.204313590394393,
-0.140848846060268));
#36751=CARTESIAN_POINT('Ctrl Pts',(0.0855901404449638,0.176014531190619,
-0.144555394640801));
#36752=CARTESIAN_POINT('Ctrl Pts',(0.143786629704924,0.147715471986845,
-0.148261943221334));
#36753=CARTESIAN_POINT('Ctrl Pts',(0.186558271156478,0.0876953018690344,
-0.151968491801868));
#36754=CARTESIAN_POINT('Ctrl Pts',(0.194311404643603,0.0234491932800436,
-0.155675040382401));
#36755=CARTESIAN_POINT('Ctrl Pts',(0.202064538130729,-0.0407969153089472,
-0.159381588962934));
#36756=CARTESIAN_POINT('Ctrl Pts',(0.174799163653426,-0.109268962369118,
-0.163088137543468));
#36757=CARTESIAN_POINT('Ctrl Pts',(0.125005521700484,-0.150600126566253,
-0.166794686124001));
#36758=CARTESIAN_POINT('Ctrl Pts',(0.0752118797475406,-0.191931290763389,
-0.170501234704534));
#36759=CARTESIAN_POINT('Ctrl Pts',(0.00288997031895642,-0.206121572097488,
-0.174207783285068));
#36760=CARTESIAN_POINT('Ctrl Pts',(-0.0588297497046916,-0.186670415188142,
-0.177914331865601));
#36761=CARTESIAN_POINT('Ctrl Pts',(-0.120549469728339,-0.167219258278796,
-0.181620880446135));
#36762=CARTESIAN_POINT('Ctrl Pts',(-0.17166700034705,-0.114126663126006,
-0.185327429026668));
#36763=CARTESIAN_POINT('Ctrl Pts',(-0.188765521256956,-0.0517142228464369,
-0.189033977607201));
#36764=CARTESIAN_POINT('Ctrl Pts',(-0.193346368909845,-0.0349933683308803,
-0.190026995333993));
#36765=CARTESIAN_POINT('Ctrl Pts',(-0.195485494223524,-0.0176035797623098,
-0.191020013060785));
#36766=CARTESIAN_POINT('Ctrl Pts',(-0.195331947549774,-0.000176736735444216,
-0.192013030787576));
#36767=CARTESIAN_POINT('Ctrl Pts',(-0.195362592747278,-0.00017879229733782,
-0.202186969212423));
#36768=CARTESIAN_POINT('Ctrl Pts',(-0.195510572130406,-0.0165602229558212,
-0.201253148343214));
#36769=CARTESIAN_POINT('Ctrl Pts',(-0.193622426540463,-0.0329080252349692,
-0.200319327474004));
#36770=CARTESIAN_POINT('Ctrl Pts',(-0.189565844057378,-0.0486987641605954,
-0.199385506604795));
#36771=CARTESIAN_POINT('Ctrl Pts',(-0.17346434050325,-0.111375818058419,
-0.195678958024261));
#36772=CARTESIAN_POINT('Ctrl Pts',(-0.123199598663687,-0.165276463407468,
-0.191972409443728));
#36773=CARTESIAN_POINT('Ctrl Pts',(-0.0617977680446978,-0.185708952011097,
-0.188265860863195));
#36774=CARTESIAN_POINT('Ctrl Pts',(-0.000395937425709474,-0.206141440614726,
-0.184559312282662));
#36775=CARTESIAN_POINT('Ctrl Pts',(0.0721429819727052,-0.193105772472937,
-0.180852763702128));
#36776=CARTESIAN_POINT('Ctrl Pts',(0.122589101633872,-0.15257355742187,
-0.177146215121595));
#36777=CARTESIAN_POINT('Ctrl Pts',(0.17303522129504,-0.112041342370802,
-0.173439666541061));
#36778=CARTESIAN_POINT('Ctrl Pts',(0.20138854121896,-0.0440125804104571,
-0.169733117960528));
#36779=CARTESIAN_POINT('Ctrl Pts',(0.194660473879366,0.0203489363561378,
-0.166026569379995));
#36780=CARTESIAN_POINT('Ctrl Pts',(0.187932406539773,0.0847104531227328,
-0.162320020799461));
#36781=CARTESIAN_POINT('Ctrl Pts',(0.146122951936665,0.145404724695577,
-0.158613472218928));
#36782=CARTESIAN_POINT('Ctrl Pts',(0.0883849226421938,0.174627847866996,
-0.154906923638395));
#36783=CARTESIAN_POINT('Ctrl Pts',(0.0306468933477237,0.203850971038415,
-0.151200375057861));
#36784=CARTESIAN_POINT('Ctrl Pts',(-0.0430197106381098,0.201602945808412,
-0.147493826477328));
#36785=CARTESIAN_POINT('Ctrl Pts',(-0.0988684271343803,0.168913614382175,
-0.143787277896795));
#36786=CARTESIAN_POINT('Ctrl Pts',(-0.154717143630652,0.136224282955937,
-0.140080729316261));
#36787=CARTESIAN_POINT('Ctrl Pts',(-0.19274797263736,0.0730936453334647,
-0.136374180735728));
#36788=CARTESIAN_POINT('Ctrl Pts',(-0.195539054829503,0.0084416304927417,
-0.132667632155194));
#36789=CARTESIAN_POINT('Ctrl Pts',(-0.195659703437486,0.0056469526377488,
-0.132507411174271));
#36790=CARTESIAN_POINT('Ctrl Pts',(-0.195714505626837,0.00284943204833622,
-0.132347190193347));
#36791=CARTESIAN_POINT('Ctrl Pts',(-0.195704662017859,5.15171773276178E-5,
-0.132186969212423));
#36792=CARTESIAN_POINT('Origin',(0.,0.,-0.56));
#36793=CARTESIAN_POINT('',(-0.195233177397639,0.000155192514023357,-0.0520130307875762));
#36794=CARTESIAN_POINT('',(-0.195209575558751,0.00014773333329694,-0.0621869692124235));
#36795=CARTESIAN_POINT('',(-0.1954,-2.39295984553393E-17,-0.56));
#36796=CARTESIAN_POINT('Ctrl Pts',(-0.195233177397639,0.000155192514023357,
-0.0520130307875762));
#36797=CARTESIAN_POINT('Ctrl Pts',(-0.195394113464411,0.0211568636252984,
-0.053208096761051));
#36798=CARTESIAN_POINT('Ctrl Pts',(-0.192275975482653,0.0421126137721153,
-0.0544031627345257));
#36799=CARTESIAN_POINT('Ctrl Pts',(-0.185678101019284,0.0619073340238181,
-0.0555982287080004));
#36800=CARTESIAN_POINT('Ctrl Pts',(-0.165214509243147,0.1233015113157,-0.0593047772885337));
#36801=CARTESIAN_POINT('Ctrl Pts',(-0.111277350974912,0.17352708098491,
-0.0630113258690671));
#36802=CARTESIAN_POINT('Ctrl Pts',(-0.0485892744020614,0.189591048794179,
-0.0667178744496004));
#36803=CARTESIAN_POINT('Ctrl Pts',(0.0140988021707893,0.205655016603449,
-0.0704244230301338));
#36804=CARTESIAN_POINT('Ctrl Pts',(0.0855377970482562,0.187557382552778,
-0.0741309716106672));
#36805=CARTESIAN_POINT('Ctrl Pts',(0.133009133465254,0.143580642561344,
-0.0778375201912005));
#36806=CARTESIAN_POINT('Ctrl Pts',(0.180480469882252,0.0996039025699099,
-0.0815440687717339));
#36807=CARTESIAN_POINT('Ctrl Pts',(0.20398414783878,0.029748056637711,-0.0852506173522672));
#36808=CARTESIAN_POINT('Ctrl Pts',(0.192749285658678,-0.0339819211704,-0.0889571659328006));
#36809=CARTESIAN_POINT('Ctrl Pts',(0.181514423478577,-0.0977118989785101,
-0.0926637145133339));
#36810=CARTESIAN_POINT('Ctrl Pts',(0.135541021161846,-0.155316008662532,
-0.0963702630938673));
#36811=CARTESIAN_POINT('Ctrl Pts',(0.0758914272689859,-0.180408157931856,
-0.100076811674401));
#36812=CARTESIAN_POINT('Ctrl Pts',(0.0162418333761251,-0.205500307201181,
-0.103783360254934));
#36813=CARTESIAN_POINT('Ctrl Pts',(-0.0570839520928653,-0.198080496055805,
-0.107489908835468));
#36814=CARTESIAN_POINT('Ctrl Pts',(-0.110496654190512,-0.161546564858329,
-0.111196457416001));
#36815=CARTESIAN_POINT('Ctrl Pts',(-0.162453562228678,-0.12600838706628,
-0.114801981873193));
#36816=CARTESIAN_POINT('Ctrl Pts',(-0.195568079320075,-0.0629215056474345,
-0.118407506330385));
#36817=CARTESIAN_POINT('Ctrl Pts',(-0.195714505993407,3.28936632279162E-5,
-0.122013030787576));
#36818=CARTESIAN_POINT('Ctrl Pts',(-0.195704662017859,5.15171773276178E-5,
-0.132186969212423));
#36819=CARTESIAN_POINT('Ctrl Pts',(-0.195486783797436,-0.0618774678483191,
-0.128640641612814));
#36820=CARTESIAN_POINT('Ctrl Pts',(-0.163598090938826,-0.123999616539142,
-0.125094314013204));
#36821=CARTESIAN_POINT('Ctrl Pts',(-0.113057776887832,-0.159764585797867,
-0.121547986413594));
#36822=CARTESIAN_POINT('Ctrl Pts',(-0.0602340813764411,-0.197145395188781,
-0.117841437833061));
#36823=CARTESIAN_POINT('Ctrl Pts',(0.0129646450239196,-0.205733621911635,
-0.114134889252528));
#36824=CARTESIAN_POINT('Ctrl Pts',(0.0730063821891976,-0.181595212509884,
-0.110428340671994));
#36825=CARTESIAN_POINT('Ctrl Pts',(0.133048119354474,-0.157456803108133,
-0.106721792091461));
#36826=CARTESIAN_POINT('Ctrl Pts',(0.179932867284669,-0.10059175758178,
-0.103015243510927));
#36827=CARTESIAN_POINT('Ctrl Pts',(0.192182602645457,-0.0370494424593577,
-0.0993086949303943));
#36828=CARTESIAN_POINT('Ctrl Pts',(0.204432338006246,0.0264928726630671,
-0.0956021463498609));
#36829=CARTESIAN_POINT('Ctrl Pts',(0.182047060797625,0.0967124573815599,
-0.0918955977693276));
#36830=CARTESIAN_POINT('Ctrl Pts',(0.13528186872857,0.141441209413879,-0.0881890491887942));
#36831=CARTESIAN_POINT('Ctrl Pts',(0.0885166766595161,0.186169961446195,
-0.0844825006082609));
#36832=CARTESIAN_POINT('Ctrl Pts',(0.0173715697300292,0.205407880792338,
-0.0807759520277275));
#36833=CARTESIAN_POINT('Ctrl Pts',(-0.0455629389330441,0.190343444572713,
-0.0770694034471942));
#36834=CARTESIAN_POINT('Ctrl Pts',(-0.10849744759612,0.175279008353088,
-0.0733628548666607));
#36835=CARTESIAN_POINT('Ctrl Pts',(-0.163221357992783,0.125912216567692,
-0.0696563062861274));
#36836=CARTESIAN_POINT('Ctrl Pts',(-0.184664120209359,0.0648553589225613,
-0.065949757705594));
#36837=CARTESIAN_POINT('Ctrl Pts',(-0.191920158828329,0.0441942653306371,
-0.0646954948745371));
#36838=CARTESIAN_POINT('Ctrl Pts',(-0.195365223212996,0.0221945598750925,
-0.0634412320434803));
#36839=CARTESIAN_POINT('Ctrl Pts',(-0.195209575558751,0.00014773333329694,
-0.0621869692124235));
#36840=CARTESIAN_POINT('Origin',(0.,0.,-1.18400562256037));
#36841=CARTESIAN_POINT('',(-0.155417199305029,0.000123542454221778,-0.0290056225603694));
#36842=CARTESIAN_POINT('',(-0.155328879770405,-0.00016163609193072,-0.0151943774396288));
#36843=CARTESIAN_POINT('',(-0.15555,-1.32567133817862E-14,-1.18400562256037));
#36844=CARTESIAN_POINT('',(0.133820452603638,-0.0798000960230315,1.68903200041158E-16));
#36845=CARTESIAN_POINT('Ctrl Pts',(-0.155417199305029,0.000123542454221769,
-0.0290056225603694));
#36846=CARTESIAN_POINT('Ctrl Pts',(-0.15514796082327,-0.0350112670250425,
-0.0264941399533108));
#36847=CARTESIAN_POINT('Ctrl Pts',(-0.125938607687929,-0.122399182856573,
-0.020276108765719));
#36848=CARTESIAN_POINT('Ctrl Pts',(0.0152304203843597,-0.181290024202016,
-0.0106075679122624));
#36849=CARTESIAN_POINT('Ctrl Pts',(0.109031119236811,-0.120890131481052,
-0.00345050966586446));
#36850=CARTESIAN_POINT('Ctrl Pts',(0.133822070517494,-0.0798006560480846,
1.69216854070675E-16));
#36851=CARTESIAN_POINT('',(-0.0319621170202048,-0.15223082991164,0.));
#36852=CARTESIAN_POINT('Origin',(0.,0.,0.));
#36853=CARTESIAN_POINT('Ctrl Pts',(-0.155328879770405,-0.000161636091930716,
-0.0151943774396288));
#36854=CARTESIAN_POINT('Ctrl Pts',(-0.155437349196103,-0.0191858047064336,
-0.0138361335402858));
#36855=CARTESIAN_POINT('Ctrl Pts',(-0.143394445718357,-0.0899409694934188,
-0.00877134106040959));
#36856=CARTESIAN_POINT('Ctrl Pts',(-0.0826091653404253,-0.141597064818995,
-0.00370654858053334));
#36857=CARTESIAN_POINT('Ctrl Pts',(-0.0319621170202048,-0.15223082991164,
0.));
#36858=CARTESIAN_POINT('Origin',(0.,0.,-1.18400562256037));
#36859=CARTESIAN_POINT('',(-0.155800365441527,2.61853086679489E-5,-0.0990056225603694));
#36860=CARTESIAN_POINT('',(-0.155398410840142,0.000117604503539592,-0.0851943774396291));
#36861=CARTESIAN_POINT('',(-0.15555,-1.32567133817862E-14,-1.18400562256037));
#36862=CARTESIAN_POINT('Ctrl Pts',(-0.155800365441527,2.61853086679508E-5,
-0.0990056225603694));
#36863=CARTESIAN_POINT('Ctrl Pts',(-0.155683801116874,-0.0500892538559854,
-0.0954000981031777));
#36864=CARTESIAN_POINT('Ctrl Pts',(-0.102222939106085,-0.151938211910091,
-0.0880880250654528));
#36865=CARTESIAN_POINT('Ctrl Pts',(0.0713011418186189,-0.169497054292766,
-0.0770694034471942));
#36866=CARTESIAN_POINT('Ctrl Pts',(0.181093814239817,-0.0319281812935353,
-0.065949757705594));
#36867=CARTESIAN_POINT('Ctrl Pts',(0.124962845363592,0.134900019854162,
-0.0548301119639941));
#36868=CARTESIAN_POINT('Ctrl Pts',(-0.045646197418241,0.178120393087247,
-0.0437104662223939));
#36869=CARTESIAN_POINT('Ctrl Pts',(-0.145364369674128,0.0852641476206765,
-0.0351023030878524));
#36870=CARTESIAN_POINT('Ctrl Pts',(-0.155545313968215,0.0168421194314946,
-0.0302006885338442));
#36871=CARTESIAN_POINT('Ctrl Pts',(-0.155417199305029,0.000123542454221769,
-0.0290056225603694));
#36872=CARTESIAN_POINT('Ctrl Pts',(-0.155398410840142,0.00011760450353957,
-0.0851943774396291));
#36873=CARTESIAN_POINT('Ctrl Pts',(-0.155156157062649,-0.0341966101071686,
-0.0827420916901529));
#36874=CARTESIAN_POINT('Ctrl Pts',(-0.127029144573819,-0.120735747049266,
-0.0765832573601433));
#36875=CARTESIAN_POINT('Ctrl Pts',(0.0160916033347015,-0.183170692569655,
-0.0667178744496004));
#36876=CARTESIAN_POINT('Ctrl Pts',(0.16268430194739,-0.0857519355616629,
-0.0555982287080002));
#36877=CARTESIAN_POINT('Ctrl Pts',(0.160190409020898,0.0902865901057441,
-0.0444785829664002));
#36878=CARTESIAN_POINT('Ctrl Pts',(0.0109996935541243,0.183501383580361,
-0.0333589372248001));
#36879=CARTESIAN_POINT('Ctrl Pts',(-0.12893036588142,0.117918227652547,
-0.023597535382543));
#36880=CARTESIAN_POINT('Ctrl Pts',(-0.155141344041178,0.0327297645135169,
-0.0175426821208192));
#36881=CARTESIAN_POINT('Ctrl Pts',(-0.155328879770405,-0.000161636091930716,
-0.0151943774396288));
#36882=CARTESIAN_POINT('Origin',(0.,0.,-1.18400562256037));
#36883=CARTESIAN_POINT('',(-0.155495826209659,-0.00014069293346625,-0.16900562256037));
#36884=CARTESIAN_POINT('',(-0.1557925290526,4.10107314749147E-5,-0.155194377439629));
#36885=CARTESIAN_POINT('',(-0.15555,-1.32567133817862E-14,-1.18400562256037));
#36886=CARTESIAN_POINT('Ctrl Pts',(-0.155495826209659,-0.000140692933466274,
-0.16900562256037));
#36887=CARTESIAN_POINT('Ctrl Pts',(-0.155618058477324,-0.0140134945344324,
-0.168012604833578));
#36888=CARTESIAN_POINT('Ctrl Pts',(-0.147559034213969,-0.0795284632520187,
-0.163313038526253));
#36889=CARTESIAN_POINT('Ctrl Pts',(-0.0552719453863964,-0.175381314233795,
-0.154906923638395));
#36890=CARTESIAN_POINT('Ctrl Pts',(0.117445654587239,-0.141492395172598,
-0.143787277896795));
#36891=CARTESIAN_POINT('Ctrl Pts',(0.182560224698972,0.0220310478193626,
-0.132667632155195));
#36892=CARTESIAN_POINT('Ctrl Pts',(0.0804139274452977,0.165369903425689,
-0.121547986413595));
#36893=CARTESIAN_POINT('Ctrl Pts',(-0.0954069371552854,0.157197434487125,
-0.110428340671994));
#36894=CARTESIAN_POINT('Ctrl Pts',(-0.155150166767694,0.054351096265153,
-0.102914219387586));
#36895=CARTESIAN_POINT('Ctrl Pts',(-0.155803631487522,0.00143038277497305,
-0.0991066466837111));
#36896=CARTESIAN_POINT('Ctrl Pts',(-0.155800365441527,2.61853086679508E-5,
-0.0990056225603694));
#36897=CARTESIAN_POINT('Ctrl Pts',(-0.1557925290526,4.10107314749112E-5,
-0.155194377439629));
#36898=CARTESIAN_POINT('Ctrl Pts',(-0.155619085054709,-0.0492581377881695,
-0.15164804984002));
#36899=CARTESIAN_POINT('Ctrl Pts',(-0.103701607366211,-0.150398227879575,
-0.144395173659877));
#36900=CARTESIAN_POINT('Ctrl Pts',(0.0685911587771073,-0.170612914816246,
-0.133435748899201));
#36901=CARTESIAN_POINT('Ctrl Pts',(0.180560286830463,-0.0348090586500559,
-0.122316103157601));
#36902=CARTESIAN_POINT('Ctrl Pts',(0.127100258123179,0.132887815499814,
-0.111196457416001));
#36903=CARTESIAN_POINT('Ctrl Pts',(-0.0428069278985511,0.17883139309898,
-0.100076811674401));
#36904=CARTESIAN_POINT('Ctrl Pts',(-0.144675382459758,0.0869352045888443,
-0.0914094516822767));
#36905=CARTESIAN_POINT('Ctrl Pts',(-0.155522315613008,0.0176681872495837,
-0.0864486402706862));
#36906=CARTESIAN_POINT('Ctrl Pts',(-0.155398410840142,0.00011760450353957,
-0.0851943774396291));
#36907=CARTESIAN_POINT('Origin',(0.,0.,-1.18400562256037));
#36908=CARTESIAN_POINT('',(-0.155310939100384,5.26711416314951E-5,-0.23900562256037));
#36909=CARTESIAN_POINT('',(-0.155520221606136,-0.000142329282771692,-0.225194377439629));
#36910=CARTESIAN_POINT('',(-0.15555,-1.32567133817862E-14,-1.18400562256037));
#36911=CARTESIAN_POINT('Ctrl Pts',(-0.155310939100384,5.2671141631511E-5,
-0.23900562256037));
#36912=CARTESIAN_POINT('Ctrl Pts',(-0.155222147753012,-0.029191772188182,
-0.236918562983445));
#36913=CARTESIAN_POINT('Ctrl Pts',(-0.133225757910032,-0.110497290353548,
-0.231124954825986));
#36914=CARTESIAN_POINT('Ctrl Pts',(-0.00196700844525682,-0.183874200155875,
-0.221624798087995));
#36915=CARTESIAN_POINT('Ctrl Pts',(0.153469544695492,-0.101295059840545,
-0.210505152346395));
#36916=CARTESIAN_POINT('Ctrl Pts',(0.168298097102307,0.074090088224943,
-0.199385506604795));
#36917=CARTESIAN_POINT('Ctrl Pts',(0.0289328015296395,0.181594284112427,
-0.188265860863195));
#36918=CARTESIAN_POINT('Ctrl Pts',(-0.122127581727067,0.12798013767017,
-0.178139232848387));
#36919=CARTESIAN_POINT('Ctrl Pts',(-0.155161813008602,0.0377682729957565,
-0.171719153414111));
#36920=CARTESIAN_POINT('Ctrl Pts',(-0.155495826209659,-0.000140692933466274,
-0.16900562256037));
#36921=CARTESIAN_POINT('Ctrl Pts',(-0.155520221606136,-0.00014232928277169,
-0.225194377439629));
#36922=CARTESIAN_POINT('Ctrl Pts',(-0.155638021979962,-0.0131829205771748,
-0.22426055657042));
#36923=CARTESIAN_POINT('Ctrl Pts',(-0.148168893704103,-0.0778515737263976,
-0.219620187120677));
#36924=CARTESIAN_POINT('Ctrl Pts',(-0.0580604758392629,-0.174477990107862,
-0.211273269090402));
#36925=CARTESIAN_POINT('Ctrl Pts',(0.115175382590983,-0.143346492982138,
-0.200153623348801));
#36926=CARTESIAN_POINT('Ctrl Pts',(0.182888160188203,0.0191183062440436,
-0.189033977607201));
#36927=CARTESIAN_POINT('Ctrl Pts',(0.0830397364904521,0.164067036179902,
-0.177914331865601));
#36928=CARTESIAN_POINT('Ctrl Pts',(-0.0928892335709049,0.158698351565871,
-0.166794686124001));
#36929=CARTESIAN_POINT('Ctrl Pts',(-0.154747501165264,0.0560145032920222,
-0.15922136798201));
#36930=CARTESIAN_POINT('Ctrl Pts',(-0.155800365149716,0.00226831706815041,
-0.155354598420553));
#36931=CARTESIAN_POINT('Ctrl Pts',(-0.1557925290526,4.10107314749112E-5,
-0.155194377439629));
#36932=CARTESIAN_POINT('Origin',(0.,0.,-1.18400562256037));
#36933=CARTESIAN_POINT('',(-0.155689062743399,0.000115235607110945,-0.30900562256037));
#36934=CARTESIAN_POINT('',(-0.155303570745334,3.97412498162469E-5,-0.295194377439629));
#36935=CARTESIAN_POINT('',(-0.15555,-1.32567133817862E-14,-1.18400562256037));
#36936=CARTESIAN_POINT('Ctrl Pts',(-0.155689062743399,0.000115235607110934,
-0.30900562256037));
#36937=CARTESIAN_POINT('Ctrl Pts',(-0.155321871925874,-0.0441841658980628,
-0.305824521133312));
#36938=CARTESIAN_POINT('Ctrl Pts',(-0.112320239215782,-0.140723170785617,
-0.29893687112572));
#36939=CARTESIAN_POINT('Ctrl Pts',(0.0515074258588442,-0.176523583699745,
-0.288342672537596));
#36940=CARTESIAN_POINT('Ctrl Pts',(0.176269718137531,-0.0523696188850282,
-0.277223026795995));
#36941=CARTESIAN_POINT('Ctrl Pts',(0.139534607376368,0.119765119560166,
-0.266103381054396));
#36942=CARTESIAN_POINT('Ctrl Pts',(-0.0250413882421251,0.182171675645894,
-0.254983735312795));
#36943=CARTESIAN_POINT('Ctrl Pts',(-0.140091288211346,0.0972868755983294,
-0.24595114914812));
#36944=CARTESIAN_POINT('Ctrl Pts',(-0.155379838240722,0.0227453891229129,
-0.240625111563978));
#36945=CARTESIAN_POINT('Ctrl Pts',(-0.155310939100384,5.2671141631511E-5,
-0.23900562256037));
#36946=CARTESIAN_POINT('Ctrl Pts',(-0.155303570745334,3.97412498162556E-5,
-0.295194377439629));
#36947=CARTESIAN_POINT('Ctrl Pts',(-0.155238650751531,-0.028378580856813,
-0.293166514720287));
#36948=CARTESIAN_POINT('Ctrl Pts',(-0.134159631932849,-0.10882985390664,
-0.287432103420411));
#36949=CARTESIAN_POINT('Ctrl Pts',(-0.00489767969399011,-0.183819477000074,
-0.277991143540001));
#36950=CARTESIAN_POINT('Ctrl Pts',(0.151835415403586,-0.103728462705588,
-0.266871497798402));
#36951=CARTESIAN_POINT('Ctrl Pts',(0.169457689254605,0.0713980317726476,
-0.255751852056801));
#36952=CARTESIAN_POINT('Ctrl Pts',(0.0318237052925425,0.181110019726059,
-0.244632206315202));
#36953=CARTESIAN_POINT('Ctrl Pts',(-0.120960013984837,0.129611271034686,
-0.23444638144281));
#36954=CARTESIAN_POINT('Ctrl Pts',(-0.155170445357094,0.0385781684553703,
-0.227967105150953));
#36955=CARTESIAN_POINT('Ctrl Pts',(-0.155520221606136,-0.00014232928277169,
-0.225194377439629));
#36956=CARTESIAN_POINT('Origin',(0.,0.,-1.18400562256037));
#36957=CARTESIAN_POINT('',(-0.155672476465762,-0.000121209602746091,-0.37900562256037));
#36958=CARTESIAN_POINT('',(-0.155666155856283,0.000123253288390569,-0.365194377439629));
#36959=CARTESIAN_POINT('',(-0.15555,-1.32567133817862E-14,-1.18400562256037));
#36960=CARTESIAN_POINT('Ctrl Pts',(-0.155672476465762,-0.000121209602746106,
-0.37900562256037));
#36961=CARTESIAN_POINT('Ctrl Pts',(-0.155740414797244,-0.0080415446494063,
-0.378437027863712));
#36962=CARTESIAN_POINT('Ctrl Pts',(-0.151588537816422,-0.067521436921519,
-0.374161884586521));
#36963=CARTESIAN_POINT('Ctrl Pts',(-0.0749118080055823,-0.167933949932374,
-0.366180192728796));
#36964=CARTESIAN_POINT('Ctrl Pts',(0.100543725038754,-0.153962819777854,
-0.355060546987196));
#36965=CARTESIAN_POINT('Ctrl Pts',(0.183881617795998,0.00106824867117576,
-0.343940901245595));
#36966=CARTESIAN_POINT('Ctrl Pts',(0.0987481244286207,0.155120593218137,
-0.332821255503996));
#36967=CARTESIAN_POINT('Ctrl Pts',(-0.0768578892449788,0.167052253441001,
-0.321701609762395));
#36968=CARTESIAN_POINT('Ctrl Pts',(-0.151954637124841,0.0663032413753942,
-0.313763065447854));
#36969=CARTESIAN_POINT('Ctrl Pts',(-0.155749714493831,0.0074325107570195,
-0.309531069713845));
#36970=CARTESIAN_POINT('Ctrl Pts',(-0.155689062743399,0.000115235607110934,
-0.30900562256037));
#36971=CARTESIAN_POINT('Ctrl Pts',(-0.155666155856283,0.00012325328839057,
-0.365194377439629));
#36972=CARTESIAN_POINT('Ctrl Pts',(-0.155289020277978,-0.0433684186858502,
-0.362072472870154));
#36973=CARTESIAN_POINT('Ctrl Pts',(-0.113636956063751,-0.139129528685827,
-0.355244019720144));
#36974=CARTESIAN_POINT('Ctrl Pts',(0.0486871260286323,-0.177322167638905,
-0.344709017989602));
#36975=CARTESIAN_POINT('Ctrl Pts',(0.175412553298172,-0.0551726700606049,
-0.333589372248002));
#36976=CARTESIAN_POINT('Ctrl Pts',(0.141425907488028,0.117525742149486,
-0.322469726506402));
#36977=CARTESIAN_POINT('Ctrl Pts',(-0.0221344224967506,0.182547677935732,
-0.311350080764802));
#36978=CARTESIAN_POINT('Ctrl Pts',(-0.139285522744779,0.0989633204492847,
-0.302258297742544));
#36979=CARTESIAN_POINT('Ctrl Pts',(-0.155357312191768,0.023564724013264,
-0.29687306330082));
#36980=CARTESIAN_POINT('Ctrl Pts',(-0.155303570745334,3.97412498162556E-5,
-0.295194377439629));
#36981=CARTESIAN_POINT('Origin',(0.,0.,-1.18400562256037));
#36982=CARTESIAN_POINT('',(-0.155305368154442,-4.32865829287516E-5,-0.44900562256037));
#36983=CARTESIAN_POINT('',(-0.155695065503602,-0.00011283858791146,-0.435194377439629));
#36984=CARTESIAN_POINT('',(-0.15555,-1.32567133817862E-14,-1.18400562256037));
#36985=CARTESIAN_POINT('Ctrl Pts',(-0.155305368154442,-4.32865829287695E-5,
-0.44900562256037));
#36986=CARTESIAN_POINT('Ctrl Pts',(-0.15536338193547,-0.023342686153529,
-0.447342986013579));
#36987=CARTESIAN_POINT('Ctrl Pts',(-0.139505759847756,-0.098508885666548,
-0.441973800886254));
#36988=CARTESIAN_POINT('Ctrl Pts',(-0.0229231396891714,-0.182450322513706,
-0.432898067178396));
#36989=CARTESIAN_POINT('Ctrl Pts',(0.140916678082541,-0.118135855508594,
-0.421778421436797));
#36990=CARTESIAN_POINT('Ctrl Pts',(0.175649365031236,0.0544140706314786,
-0.410658775695196));
#36991=CARTESIAN_POINT('Ctrl Pts',(0.0494530132129136,0.177110107003317,
-0.399539129953596));
#36992=CARTESIAN_POINT('Ctrl Pts',(-0.113282157194832,0.139562230312325,
-0.388988078908654));
#36993=CARTESIAN_POINT('Ctrl Pts',(-0.155297539181982,0.0435894445193366,
-0.382143576444245));
#36994=CARTESIAN_POINT('Ctrl Pts',(-0.155672476465762,-0.000121209602746106,
-0.37900562256037));
#36995=CARTESIAN_POINT('Ctrl Pts',(-0.155695065503602,-0.000112838587911464,
-0.435194377439629));
#36996=CARTESIAN_POINT('Ctrl Pts',(-0.155752997892932,-0.00720589989722735,
-0.434684979600554));
#36997=CARTESIAN_POINT('Ctrl Pts',(-0.152088815062267,-0.0658502493267181,
-0.430469033180945));
#36998=CARTESIAN_POINT('Ctrl Pts',(-0.0775791235918538,-0.166718526143494,
-0.422546538180803));
#36999=CARTESIAN_POINT('Ctrl Pts',(0.098076807463925,-0.1555459006674,-0.411426892439203));
#37000=CARTESIAN_POINT('Ctrl Pts',(0.183875275341805,-0.00186292638295208,
-0.400307246697602));
#37001=CARTESIAN_POINT('Ctrl Pts',(0.101208168018179,0.153526851407609,
-0.389187600956003));
#37002=CARTESIAN_POINT('Ctrl Pts',(-0.0741853388097491,0.168256122867715,
-0.378067955214402));
#37003=CARTESIAN_POINT('Ctrl Pts',(-0.151450355425137,0.0679746909538998,
-0.370070214042278));
#37004=CARTESIAN_POINT('Ctrl Pts',(-0.155736782633081,0.00826800755129776,
-0.365779021450687));
#37005=CARTESIAN_POINT('Ctrl Pts',(-0.155666155856283,0.00012325328839057,
-0.365194377439629));
#37006=CARTESIAN_POINT('Origin',(0.,0.,-1.18400562256037));
#37007=CARTESIAN_POINT('',(-0.155513557532958,0.000142022966550295,-0.51900562256037));
#37008=CARTESIAN_POINT('',(-0.155313283030358,-5.6100541927756E-5,-0.505194377439629));
#37009=CARTESIAN_POINT('',(-0.15555,-1.32567133817862E-14,-1.18400562256037));
#37010=CARTESIAN_POINT('Ctrl Pts',(-0.155513557532958,0.000142022966550288,
-0.51900562256037));
#37011=CARTESIAN_POINT('Ctrl Pts',(-0.155167810588833,-0.0383585585219179,
-0.516248944163445));
#37012=CARTESIAN_POINT('Ctrl Pts',(-0.121278654951446,-0.129169493585072,
-0.509785717185988));
#37013=CARTESIAN_POINT('Ctrl Pts',(0.0310407000630972,-0.181245870182351,
-0.499615941627997));
#37014=CARTESIAN_POINT('Ctrl Pts',(0.169147551063838,-0.0721297198640855,
-0.488496295886397));
#37015=CARTESIAN_POINT('Ctrl Pts',(0.152282291589484,0.103071306321499,
-0.477376650144796));
#37016=CARTESIAN_POINT('Ctrl Pts',(-0.00410321495424111,0.183838935336354,
-0.466257004403197));
#37017=CARTESIAN_POINT('Ctrl Pts',(-0.133908341240762,0.109282116163178,
-0.456799995208387));
#37018=CARTESIAN_POINT('Ctrl Pts',(-0.155234050664522,0.028599126729369,
-0.451049534594112));
#37019=CARTESIAN_POINT('Ctrl Pts',(-0.155305368154442,-4.32865829287695E-5,
-0.44900562256037));
#37020=CARTESIAN_POINT('Ctrl Pts',(-0.155313283030358,-5.6100541927763E-5,
-0.505194377439629));
#37021=CARTESIAN_POINT('Ctrl Pts',(-0.15538600368638,-0.0225230806948092,
-0.50359093775042));
#37022=CARTESIAN_POINT('Ctrl Pts',(-0.140306651967032,-0.096832232461837,
-0.498280949480678));
#37023=CARTESIAN_POINT('Ctrl Pts',(-0.0258284510112228,-0.182061743634136,
-0.489264412630403));
#37024=CARTESIAN_POINT('Ctrl Pts',(0.139015704615632,-0.120367027241518,
-0.478144766888803));
#37025=CARTESIAN_POINT('Ctrl Pts',(0.176494391467026,0.0516073362752325,
-0.467025121147203));
#37026=CARTESIAN_POINT('Ctrl Pts',(0.0522698307062849,0.176299325508287,
-0.455905475405603));
#37027=CARTESIAN_POINT('Ctrl Pts',(-0.111959433833773,0.141154106954363,
-0.445295227503078));
#37028=CARTESIAN_POINT('Ctrl Pts',(-0.155331462505528,0.0444055799932159,
-0.438391528181087));
#37029=CARTESIAN_POINT('Ctrl Pts',(-0.155695065503602,-0.000112838587911464,
-0.435194377439629));
#37030=CARTESIAN_POINT('Origin',(0.,0.,-1.18400562256037));
#37031=CARTESIAN_POINT('',(-0.155794948693578,-3.70111496645316E-5,-0.589005622560369));
#37032=CARTESIAN_POINT('',(-0.15548930789199,0.000140015377334053,-0.575194377439629));
#37033=CARTESIAN_POINT('',(-0.15555,-1.32567133817862E-14,-1.18400562256037));
#37034=CARTESIAN_POINT('Ctrl Pts',(-0.155794948693578,-3.70111496645414E-5,
-0.58900562256037));
#37035=CARTESIAN_POINT('Ctrl Pts',(-0.155801375060938,-0.00204112484285652,
-0.588861450893845));
#37036=CARTESIAN_POINT('Ctrl Pts',(-0.15485797915675,-0.0555633522856045,
-0.585010730646788));
#37037=CARTESIAN_POINT('Ctrl Pts',(-0.0935742393001708,-0.15829545874079,
-0.577453461819198));
#37038=CARTESIAN_POINT('Ctrl Pts',(0.0823299191069159,-0.164424374526445,
-0.566333816077597));
#37039=CARTESIAN_POINT('Ctrl Pts',(0.182803831914859,-0.0199085297249743,
-0.555214170335998));
#37040=CARTESIAN_POINT('Ctrl Pts',(0.115793820441273,0.142847406928437,
-0.544094524594397));
#37041=CARTESIAN_POINT('Ctrl Pts',(-0.057305889765134,0.174727288987128,
-0.532974878852797));
#37042=CARTESIAN_POINT('Ctrl Pts',(-0.148005123032518,0.0783061562763419,
-0.524611911508121));
#37043=CARTESIAN_POINT('Ctrl Pts',(-0.155632691746678,0.0134081893965227,
-0.519955492743979));
#37044=CARTESIAN_POINT('Ctrl Pts',(-0.155513557532958,0.000142022966550288,
-0.51900562256037));
#37045=CARTESIAN_POINT('Ctrl Pts',(-0.15548930789199,0.000140015377334046,
-0.575194377439629));
#37046=CARTESIAN_POINT('Ctrl Pts',(-0.155159975094503,-0.037548743133565,
-0.572496895900287));
#37047=CARTESIAN_POINT('Ctrl Pts',(-0.122440493891221,-0.127537141042073,
-0.566092865780412));
#37048=CARTESIAN_POINT('Ctrl Pts',(0.028147729041889,-0.181717618096114,
-0.555982287080003));
#37049=CARTESIAN_POINT('Ctrl Pts',(0.167976319009287,-0.0748167336150888,
-0.544862641338404));
#37050=CARTESIAN_POINT('Ctrl Pts',(0.153905875245583,0.100630854819146,
-0.533742995596803));
#37051=CARTESIAN_POINT('Ctrl Pts',(-0.00117233452664475,0.183880975112975,
-0.522623349855203));
#37052=CARTESIAN_POINT('Ctrl Pts',(-0.132969246133086,0.11094901835971,
-0.513107143802813));
#37053=CARTESIAN_POINT('Ctrl Pts',(-0.15521790092195,0.0294121145950307,
-0.507297486330954));
#37054=CARTESIAN_POINT('Ctrl Pts',(-0.155313283030358,-5.6100541927763E-5,
-0.505194377439629));
#37055=CARTESIAN_POINT('Origin',(0.,0.,-1.18400562256037));
#37056=CARTESIAN_POINT('',(-0.15540393784838,-0.000119995988950991,-0.65900562256037));
#37057=CARTESIAN_POINT('',(-0.155801839037753,-2.20116907670709E-5,-0.645194377439629));
#37058=CARTESIAN_POINT('',(-0.15555,-1.32567133817862E-14,-1.18400562256037));
#37059=CARTESIAN_POINT('Ctrl Pts',(-0.15540393784838,-0.000119995988950999,
-0.65900562256037));
#37060=CARTESIAN_POINT('Ctrl Pts',(-0.155528444664855,-0.0174441538003097,
-0.657767409043713));
#37061=CARTESIAN_POINT('Ctrl Pts',(-0.144860866850051,-0.0864786497960442,
-0.652822646946522));
#37062=CARTESIAN_POINT('Ctrl Pts',(-0.0435801783122908,-0.178645902770777,
-0.644171336268797));
#37063=CARTESIAN_POINT('Ctrl Pts',(0.126525183886544,-0.133435259062113,
-0.633051690527199));
#37064=CARTESIAN_POINT('Ctrl Pts',(0.180708827729641,0.0340280781002357,
-0.621932044785597));
#37065=CARTESIAN_POINT('Ctrl Pts',(0.0693279792777336,0.170315066297202,
-0.610812399043998));
#37066=CARTESIAN_POINT('Ctrl Pts',(-0.103303156215773,0.150816403206739,
-0.599836924968922));
#37067=CARTESIAN_POINT('Ctrl Pts',(-0.155636157834885,0.0494831790916029,
-0.592567999474379));
#37068=CARTESIAN_POINT('Ctrl Pts',(-0.155794948693578,-3.70111496645414E-5,
-0.58900562256037));
#37069=CARTESIAN_POINT('Ctrl Pts',(-0.155801839037753,-2.20116907670611E-5,
-0.645194377439629));
#37070=CARTESIAN_POINT('Ctrl Pts',(-0.155804177189137,-0.00120309644097989,
-0.645109402630688));
#37071=CARTESIAN_POINT('Ctrl Pts',(-0.155256813551466,-0.0539001433168381,
-0.641317879241212));
#37072=CARTESIAN_POINT('Ctrl Pts',(-0.0960855472312445,-0.156783784206156,
-0.633819807271204));
#37073=CARTESIAN_POINT('Ctrl Pts',(0.0796985611215568,-0.165715801092974,
-0.622700161529604));
#37074=CARTESIAN_POINT('Ctrl Pts',(0.182463260436913,-0.0228198590591629,
-0.611580515788004));
#37075=CARTESIAN_POINT('Ctrl Pts',(0.118056065295367,0.140983519688348,
-0.600460870046404));
#37076=CARTESIAN_POINT('Ctrl Pts',(-0.054513485600872,0.175618527679694,
-0.589341224304804));
#37077=CARTESIAN_POINT('Ctrl Pts',(-0.14739093441373,0.0799831865833066,
-0.580919060102545));
#37078=CARTESIAN_POINT('Ctrl Pts',(-0.155612503868192,0.0142385304114906,
-0.576203444480821));
#37079=CARTESIAN_POINT('Ctrl Pts',(-0.15548930789199,0.000140015377334046,
-0.575194377439629));
#37080=CARTESIAN_POINT('Origin',(0.,0.,-1.18400562256037));
#37081=CARTESIAN_POINT('',(-0.155362436352018,9.99900651833539E-5,-0.72900562256037));
#37082=CARTESIAN_POINT('',(-0.155424369060156,-0.000126926758710719,-0.715194377439629));
#37083=CARTESIAN_POINT('',(-0.15555,-1.32567133817862E-14,-1.18400562256037));
#37084=CARTESIAN_POINT('Ctrl Pts',(-0.155362436352018,9.99900651833512E-5,
-0.72900562256037));
#37085=CARTESIAN_POINT('Ctrl Pts',(-0.155170334697732,-0.032553096980618,
-0.72667336719358));
#37086=CARTESIAN_POINT('Ctrl Pts',(-0.129150367964797,-0.117380331222216,
-0.720634563246256));
#37087=CARTESIAN_POINT('Ctrl Pts',(0.0101689670613149,-0.183603329566334,
-0.710889210718397));
#37088=CARTESIAN_POINT('Ctrl Pts',(0.159818411126364,-0.0909486997130359,
-0.6997695649768));
#37089=CARTESIAN_POINT('Ctrl Pts',(0.163043054468382,0.0850326579052167,
-0.688649919235197));
#37090=CARTESIAN_POINT('Ctrl Pts',(0.0168884954843339,0.183107534631158,
-0.677530273493599));
#37091=CARTESIAN_POINT('Ctrl Pts',(-0.126741374559613,0.121180173616676,
-0.667648841268655));
#37092=CARTESIAN_POINT('Ctrl Pts',(-0.155155737892023,0.0344151028471008,
-0.661473957624246));
#37093=CARTESIAN_POINT('Ctrl Pts',(-0.15540393784838,-0.000119995988950999,
-0.65900562256037));
#37094=CARTESIAN_POINT('Ctrl Pts',(-0.155424369060156,-0.000126926758710741,
-0.715194377439629));
#37095=CARTESIAN_POINT('Ctrl Pts',(-0.155550893466124,-0.0166173779854387,
-0.714015360780554));
#37096=CARTESIAN_POINT('Ctrl Pts',(-0.145538034253706,-0.0848002269033668,
-0.709129795540946));
#37097=CARTESIAN_POINT('Ctrl Pts',(-0.0464222225043185,-0.177928537998713,
-0.700537681720804));
#37098=CARTESIAN_POINT('Ctrl Pts',(0.124382169793526,-0.135435088561476,
-0.689418035979205));
#37099=CARTESIAN_POINT('Ctrl Pts',(0.181228262157198,0.0311432877610799,
-0.678298390237604));
#37100=CARTESIAN_POINT('Ctrl Pts',(0.0720339590899123,0.169188345090688,
-0.667178744496004));
#37101=CARTESIAN_POINT('Ctrl Pts',(-0.101818695314802,0.152353556505981,
-0.656144073563346));
#37102=CARTESIAN_POINT('Ctrl Pts',(-0.155702188472728,0.0503150894650411,
-0.648815951211221));
#37103=CARTESIAN_POINT('Ctrl Pts',(-0.155801839037753,-2.20116907670611E-5,
-0.645194377439629));
#37104=CARTESIAN_POINT('Origin',(0.,0.,-1.18400562256037));
#37105=CARTESIAN_POINT('',(-0.155767789804036,6.93381960118415E-5,-0.79900562256037));
#37106=CARTESIAN_POINT('',(-0.155347070724463,8.97218886615411E-5,-0.78519437743963));
#37107=CARTESIAN_POINT('',(-0.15555,-1.32567133817862E-14,-1.18400562256037));
#37108=CARTESIAN_POINT('Ctrl Pts',(-0.155767789804036,6.93381960118404E-5,
-0.79900562256037));
#37109=CARTESIAN_POINT('Ctrl Pts',(-0.155502544361867,-0.0475813235126791,
-0.795579325343446));
#37110=CARTESIAN_POINT('Ctrl Pts',(-0.106628930778583,-0.147250628696526,
-0.78844647954599));
#37111=CARTESIAN_POINT('Ctrl Pts',(0.0630419049178878,-0.172740582625397,
-0.777607085167998));
#37112=CARTESIAN_POINT('Ctrl Pts',(0.179340890619455,-0.0406255492142766,
-0.766487439426399));
#37113=CARTESIAN_POINT('Ctrl Pts',(0.131328683099859,0.128710402067756,
-0.755367793684797));
#37114=CARTESIAN_POINT('Ctrl Pts',(-0.037006185026792,0.180122549393705,
-0.7442481479432));
#37115=CARTESIAN_POINT('Ctrl Pts',(-0.14324057853946,0.0903372148411208,
-0.735460757568388));
#37116=CARTESIAN_POINT('Ctrl Pts',(-0.155475633218705,0.0193409859585915,
-0.730379915774113));
#37117=CARTESIAN_POINT('Ctrl Pts',(-0.155362436352018,9.99900651833512E-5,
-0.72900562256037));
#37118=CARTESIAN_POINT('Ctrl Pts',(-0.155347070724463,8.9721888661529E-5,
-0.78519437743963));
#37119=CARTESIAN_POINT('Ctrl Pts',(-0.155180081869041,-0.0317424574751034,
-0.782921318930421));
#37120=CARTESIAN_POINT('Ctrl Pts',(-0.13016521763349,-0.115722480957532,
-0.776941711840679));
#37121=CARTESIAN_POINT('Ctrl Pts',(0.00724107137421544,-0.183742086289102,
-0.767255556170406));
#37122=CARTESIAN_POINT('Ctrl Pts',(0.158348393578249,-0.0934846169015645,
-0.756135910428804));
#37123=CARTESIAN_POINT('Ctrl Pts',(0.164377737792651,0.0824229744011697,
-0.745016264687206));
#37124=CARTESIAN_POINT('Ctrl Pts',(0.0198050495896289,0.182815063350545,
-0.733896618945604));
#37125=CARTESIAN_POINT('Ctrl Pts',(-0.125659926754502,0.122827779940055,
-0.72395598986308));
#37126=CARTESIAN_POINT('Ctrl Pts',(-0.155153130759608,0.0352246872782868,
-0.717721909361088));
#37127=CARTESIAN_POINT('Ctrl Pts',(-0.155424369060156,-0.000126926758710741,
-0.715194377439629));
#37128=CARTESIAN_POINT('Origin',(0.,0.,-1.18400562256037));
#37129=CARTESIAN_POINT('',(-0.155570908001796,-0.000141339127694456,-0.86900562256037));
#37130=CARTESIAN_POINT('',(-0.155751765103858,8.20881598970168E-5,-0.855194377439629));
#37131=CARTESIAN_POINT('',(-0.15555,-1.32567133817862E-14,-1.18400562256037));
#37132=CARTESIAN_POINT('Ctrl Pts',(-0.155570908001796,-0.000141339127694456,
-0.86900562256037));
#37133=CARTESIAN_POINT('Ctrl Pts',(-0.15567590648691,-0.0114962743919849,
-0.868191832073847));
#37134=CARTESIAN_POINT('Ctrl Pts',(-0.149357049078014,-0.0744533324005729,
-0.863671493006789));
#37135=CARTESIAN_POINT('Ctrl Pts',(-0.0636687064710734,-0.17251058084216,
-0.8554446053592));
#37136=CARTESIAN_POINT('Ctrl Pts',(0.110482893512257,-0.146993649357098,
-0.844324959617598));
#37137=CARTESIAN_POINT('Ctrl Pts',(0.18341044091426,0.0131980997397562,
-0.833205313875999));
#37138=CARTESIAN_POINT('Ctrl Pts',(0.0882983957762384,0.161297819676871,
-0.822085668134399));
#37139=CARTESIAN_POINT('Ctrl Pts',(-0.0877122368719845,0.161617311611651,
-0.810966022392799));
#37140=CARTESIAN_POINT('Ctrl Pts',(-0.153888977708246,0.0593911412520667,
-0.803272673868122));
#37141=CARTESIAN_POINT('Ctrl Pts',(-0.155789485352365,0.00396688767152082,
-0.79928587392398));
#37142=CARTESIAN_POINT('Ctrl Pts',(-0.155767789804036,6.93381960118404E-5,
-0.79900562256037));
#37143=CARTESIAN_POINT('Ctrl Pts',(-0.155751765103858,8.20881598970159E-5,
-0.85519437743963));
#37144=CARTESIAN_POINT('Ctrl Pts',(-0.155452044257622,-0.0467580259285011,
-0.851827277080288));
#37145=CARTESIAN_POINT('Ctrl Pts',(-0.108038257994642,-0.14568622625586,
-0.844753628140413));
#37146=CARTESIAN_POINT('Ctrl Pts',(0.060280446378822,-0.173723506052108,
-0.833973430620006));
#37147=CARTESIAN_POINT('Ctrl Pts',(0.178670530140934,-0.0434790462684611,
-0.822853784878404));
#37148=CARTESIAN_POINT('Ctrl Pts',(0.133363614212077,0.126600688351419,
-0.811734139136806));
#37149=CARTESIAN_POINT('Ctrl Pts',(-0.0341303623589111,0.180689528985939,
-0.800614493395204));
#37150=CARTESIAN_POINT('Ctrl Pts',(-0.142507620182121,0.0920156013334908,
-0.791767906162814));
#37151=CARTESIAN_POINT('Ctrl Pts',(-0.155452381197247,0.0201644858605286,
-0.786627867510955));
#37152=CARTESIAN_POINT('Ctrl Pts',(-0.155347070724463,8.9721888661529E-5,
-0.78519437743963));
#37153=CARTESIAN_POINT('Origin',(0.,0.,-1.18400562256037));
#37154=CARTESIAN_POINT('',(-0.15529890300355,1.25102102450688E-5,-0.93900562256037));
#37155=CARTESIAN_POINT('',(-0.155595980901295,-0.000138704452836119,-0.925194377439629));
#37156=CARTESIAN_POINT('',(-0.15555,-1.32567133817862E-14,-1.18400562256037));
#37157=CARTESIAN_POINT('Ctrl Pts',(-0.15529890300355,1.25102102450734E-5,
-0.93900562256037));
#37158=CARTESIAN_POINT('Ctrl Pts',(-0.155277540336578,-0.0267273135833239,
-0.937097790223713));
#37159=CARTESIAN_POINT('Ctrl Pts',(-0.135987452190703,-0.105443411679473,
-0.931483409306522));
#37160=CARTESIAN_POINT('Ctrl Pts',(-0.0108405547554956,-0.183565275721231,
-0.922162479808802));
#37161=CARTESIAN_POINT('Ctrl Pts',(0.148406703733419,-0.108580977171968,
-0.911042834067198));
#37162=CARTESIAN_POINT('Ctrl Pts',(0.171675085100322,0.0658845155887245,
-0.899923188325601));
#37163=CARTESIAN_POINT('Ctrl Pts',(0.037660590930604,0.179987027118587,
-0.888803542583998));
#37164=CARTESIAN_POINT('Ctrl Pts',(-0.118527703919238,0.132904165366808,
-0.878497687328924));
#37165=CARTESIAN_POINT('Ctrl Pts',(-0.155197672847659,0.0402217290534668,
-0.87189838065438));
#37166=CARTESIAN_POINT('Ctrl Pts',(-0.155570908001796,-0.000141339127694456,
-0.86900562256037));
#37167=CARTESIAN_POINT('Ctrl Pts',(-0.155595980901295,-0.000138704452836098,
-0.925194377439629));
#37168=CARTESIAN_POINT('Ctrl Pts',(-0.155692996261753,-0.010663309100421,
-0.924439783810688));
#37169=CARTESIAN_POINT('Ctrl Pts',(-0.149918881858646,-0.0727785826548655,
-0.919978641601213));
#37170=CARTESIAN_POINT('Ctrl Pts',(-0.0664110274107763,-0.171473678917601,
-0.911810950811206));
#37171=CARTESIAN_POINT('Ctrl Pts',(0.108126128703887,-0.148736101992464,
-0.900691305069605));
#37172=CARTESIAN_POINT('Ctrl Pts',(0.183597333320993,0.010272923727082,
-0.889571659328006));
#37173=CARTESIAN_POINT('Ctrl Pts',(0.0908583219823267,0.15986984368347,
-0.878452013586405));
#37174=CARTESIAN_POINT('Ctrl Pts',(-0.0851249865183533,0.162994896424521,
-0.867332367844806));
#37175=CARTESIAN_POINT('Ctrl Pts',(-0.153444406068025,0.0610581867156833,
-0.859579822462547));
#37176=CARTESIAN_POINT('Ctrl Pts',(-0.155781980926748,0.00480419077368596,
-0.855533825660821));
#37177=CARTESIAN_POINT('Ctrl Pts',(-0.155751765103858,8.20881598970159E-5,
-0.85519437743963));
#37178=CARTESIAN_POINT('Origin',(0.,0.,-1.18400562256037));
#37179=CARTESIAN_POINT('',(-0.15555,-1.32567133817862E-14,-1.));
#37180=CARTESIAN_POINT('',(-0.155319281545194,2.55672115835603E-6,-0.995194377439629));
#37181=CARTESIAN_POINT('',(-0.15555,-1.32567133817862E-14,-1.18400562256037));
#37182=CARTESIAN_POINT('',(-0.107438039834496,-0.112484977203719,-1.));
#37183=CARTESIAN_POINT('Origin',(0.,0.,-1.));
#37184=CARTESIAN_POINT('Ctrl Pts',(-0.107438039834496,-0.112484977203719,
-1.));
#37185=CARTESIAN_POINT('Ctrl Pts',(-0.070014397862351,-0.148229508046032,
-0.996293451419467));
#37186=CARTESIAN_POINT('Ctrl Pts',(0.0426645675892999,-0.178810969987729,
-0.988880354258401));
#37187=CARTESIAN_POINT('Ctrl Pts',(0.173668580798161,-0.0608101377048221,
-0.977760708516799));
#37188=CARTESIAN_POINT('Ctrl Pts',(0.145082536077593,0.112893009936692,
-0.9666410627752));
#37189=CARTESIAN_POINT('Ctrl Pts',(-0.016188327655916,0.183168151262569,
-0.9555214170336));
#37190=CARTESIAN_POINT('Ctrl Pts',(-0.137605454051508,0.102359736842961,
-0.946309603628658));
#37191=CARTESIAN_POINT('Ctrl Pts',(-0.155319043859408,0.0252229831075507,
-0.940804338804247));
#37192=CARTESIAN_POINT('Ctrl Pts',(-0.15529890300355,1.25102102450734E-5,
-0.93900562256037));
#37193=CARTESIAN_POINT('Ctrl Pts',(-0.155319281545194,2.55672115836644E-6,
-0.995194377439629));
#37194=CARTESIAN_POINT('Ctrl Pts',(-0.155306686282912,-0.0259101337848701,
-0.993345741960555));
#37195=CARTESIAN_POINT('Ctrl Pts',(-0.136821575085788,-0.103778540630361,
-0.987790557900947));
#37196=CARTESIAN_POINT('Ctrl Pts',(-0.0137950195410933,-0.183363935742736,
-0.978528825260807));
#37197=CARTESIAN_POINT('Ctrl Pts',(0.14667274202516,-0.110935491613379,
-0.967409179519206));
#37198=CARTESIAN_POINT('Ctrl Pts',(0.172695229799944,0.0631411111612149,
-0.956289533777606));
#37199=CARTESIAN_POINT('Ctrl Pts',(0.0405290837896907,0.179363093540042,
-0.945169888036005));
#37200=CARTESIAN_POINT('Ctrl Pts',(-0.117297335950851,0.134520793240012,
-0.934804835923348));
#37201=CARTESIAN_POINT('Ctrl Pts',(-0.155216458781444,0.0410333351873348,
-0.928146332391221));
#37202=CARTESIAN_POINT('Ctrl Pts',(-0.155595980901295,-0.000138704452836098,
-0.925194377439629));
#37203=CARTESIAN_POINT('Ctrl Pts',(0.124290537174079,0.0935289520361411,
-1.02300740822721));
#37204=CARTESIAN_POINT('Ctrl Pts',(0.0931735462474481,0.134880292271595,
-1.01930085964667));
#37205=CARTESIAN_POINT('Ctrl Pts',(-0.013037262777072,0.183367614985409,
-1.01188776248561));
#37206=CARTESIAN_POINT('Ctrl Pts',(-0.161477093702181,0.0882259055140853,
-1.00076811674401));
#37207=CARTESIAN_POINT('Ctrl Pts',(-0.161500828769186,-0.0878136284471678,
-0.989648471002406));
#37208=CARTESIAN_POINT('Ctrl Pts',(-0.0137950195410933,-0.183363935742736,
-0.978528825260807));
#37209=CARTESIAN_POINT('Ctrl Pts',(0.14667274202516,-0.110935491613379,
-0.967409179519206));
#37210=CARTESIAN_POINT('Ctrl Pts',(0.172695229799944,0.0631411111612149,
-0.956289533777606));
#37211=CARTESIAN_POINT('Ctrl Pts',(0.0405290837896907,0.179363093540042,
-0.945169888036005));
#37212=CARTESIAN_POINT('Ctrl Pts',(-0.128787370879799,0.131256196618047,
-0.934050242294407));
#37213=CARTESIAN_POINT('Ctrl Pts',(-0.180100169418625,-0.0371083441993324,
-0.922930596552805));
#37214=CARTESIAN_POINT('Ctrl Pts',(-0.0664110274107763,-0.171473678917601,
-0.911810950811206));
#37215=CARTESIAN_POINT('Ctrl Pts',(0.108126128703887,-0.148736101992464,
-0.900691305069605));
#37216=CARTESIAN_POINT('Ctrl Pts',(0.183597333320993,0.010272923727082,
-0.889571659328006));
#37217=CARTESIAN_POINT('Ctrl Pts',(0.0908583219823267,0.15986984368347,
-0.878452013586405));
#37218=CARTESIAN_POINT('Ctrl Pts',(-0.0851249865183533,0.162994896424521,
-0.867332367844806));
#37219=CARTESIAN_POINT('Ctrl Pts',(-0.183117027223152,0.016784839709399,
-0.856212722103206));
#37220=CARTESIAN_POINT('Ctrl Pts',(-0.113338298618642,-0.144803384848188,
-0.845093076361605));
#37221=CARTESIAN_POINT('Ctrl Pts',(0.060280446378822,-0.173723506052108,
-0.833973430620006));
#37222=CARTESIAN_POINT('Ctrl Pts',(0.178670530140934,-0.0434790462684611,
-0.822853784878404));
#37223=CARTESIAN_POINT('Ctrl Pts',(0.133363614212077,0.126600688351419,
-0.811734139136806));
#37224=CARTESIAN_POINT('Ctrl Pts',(-0.0341303623589111,0.180689528985939,
-0.800614493395204));
#37225=CARTESIAN_POINT('Ctrl Pts',(-0.170354273544413,0.0692315581199349,
-0.789494847653606));
#37226=CARTESIAN_POINT('Ctrl Pts',(-0.150500483525886,-0.105656007506409,
-0.778375201912004));
#37227=CARTESIAN_POINT('Ctrl Pts',(0.00724107137421544,-0.183742086289102,
-0.767255556170406));
#37228=CARTESIAN_POINT('Ctrl Pts',(0.158348393578249,-0.0934846169015645,
-0.756135910428804));
#37229=CARTESIAN_POINT('Ctrl Pts',(0.164377737792651,0.0824229744011697,
-0.745016264687206));
#37230=CARTESIAN_POINT('Ctrl Pts',(0.0198050495896289,0.182815063350545,
-0.733896618945604));
#37231=CARTESIAN_POINT('Ctrl Pts',(-0.142912922414824,0.115712937822271,
-0.722776973204005));
#37232=CARTESIAN_POINT('Ctrl Pts',(-0.174694814920481,-0.0574047821953129,
-0.711657327462404));
#37233=CARTESIAN_POINT('Ctrl Pts',(-0.0464222225043185,-0.177928537998713,
-0.700537681720804));
#37234=CARTESIAN_POINT('Ctrl Pts',(0.124382169793526,-0.135435088561476,
-0.689418035979205));
#37235=CARTESIAN_POINT('Ctrl Pts',(0.181228262157198,0.0311432877610799,
-0.678298390237604));
#37236=CARTESIAN_POINT('Ctrl Pts',(0.0720339590899123,0.169188345090688,
-0.667178744496004));
#37237=CARTESIAN_POINT('Ctrl Pts',(-0.103157484317412,0.152223916668754,
-0.656059098754404));
#37238=CARTESIAN_POINT('Ctrl Pts',(-0.183836574721314,-0.00420727602229024,
-0.644939453012804));
#37239=CARTESIAN_POINT('Ctrl Pts',(-0.0960855472312445,-0.156783784206156,
-0.633819807271204));
#37240=CARTESIAN_POINT('Ctrl Pts',(0.0796985611215568,-0.165715801092974,
-0.622700161529604));
#37241=CARTESIAN_POINT('Ctrl Pts',(0.182463260436913,-0.0228198590591629,
-0.611580515788004));
#37242=CARTESIAN_POINT('Ctrl Pts',(0.118056065295367,0.140983519688348,
-0.600460870046404));
#37243=CARTESIAN_POINT('Ctrl Pts',(-0.054513485600872,0.175618527679694,
-0.589341224304804));
#37244=CARTESIAN_POINT('Ctrl Pts',(-0.177138063248702,0.0493527499258254,
-0.578221578563203));
#37245=CARTESIAN_POINT('Ctrl Pts',(-0.137469664530806,-0.122129761772175,
-0.567101932821604));
#37246=CARTESIAN_POINT('Ctrl Pts',(0.028147729041889,-0.181717618096114,
-0.555982287080003));
#37247=CARTESIAN_POINT('Ctrl Pts',(0.167976319009287,-0.0748167336150888,
-0.544862641338404));
#37248=CARTESIAN_POINT('Ctrl Pts',(0.153905875245583,0.100630854819146,
-0.533742995596803));
#37249=CARTESIAN_POINT('Ctrl Pts',(-0.00117233452664475,0.183880975112975,
-0.522623349855203));
#37250=CARTESIAN_POINT('Ctrl Pts',(-0.155176457475656,0.0986602981043884,
-0.511503704113604));
#37251=CARTESIAN_POINT('Ctrl Pts',(-0.167008713555752,-0.0769524331856614,
-0.500384058372002));
#37252=CARTESIAN_POINT('Ctrl Pts',(-0.0258284510112228,-0.182061743634136,
-0.489264412630403));
#37253=CARTESIAN_POINT('Ctrl Pts',(0.139015704615632,-0.120367027241518,
-0.478144766888803));
#37254=CARTESIAN_POINT('Ctrl Pts',(0.176494391467026,0.0516073362752325,
-0.467025121147203));
#37255=CARTESIAN_POINT('Ctrl Pts',(0.0522698307062849,0.176299325508287,
-0.455905475405603));
#37256=CARTESIAN_POINT('Ctrl Pts',(-0.11984407830563,0.139466785550596,
-0.444785829664003));
#37257=CARTESIAN_POINT('Ctrl Pts',(-0.182157463300752,-0.0251445011995766,
-0.433666183922403));
#37258=CARTESIAN_POINT('Ctrl Pts',(-0.0775791235918538,-0.166718526143494,
-0.422546538180803));
#37259=CARTESIAN_POINT('Ctrl Pts',(0.098076807463925,-0.1555459006674,-0.411426892439203));
#37260=CARTESIAN_POINT('Ctrl Pts',(0.183875275341805,-0.00186292638295208,
-0.400307246697602));
#37261=CARTESIAN_POINT('Ctrl Pts',(0.101208168018179,0.153526851407609,
-0.389187600956003));
#37262=CARTESIAN_POINT('Ctrl Pts',(-0.0741853388097491,0.168256122867715,
-0.378067955214402));
#37263=CARTESIAN_POINT('Ctrl Pts',(-0.181610622335615,0.0288300057499716,
-0.366948309472803));
#37264=CARTESIAN_POINT('Ctrl Pts',(-0.122645194018816,-0.137010013359534,
-0.355828663731202));
#37265=CARTESIAN_POINT('Ctrl Pts',(0.0486871260286323,-0.177322167638905,
-0.344709017989602));
#37266=CARTESIAN_POINT('Ctrl Pts',(0.175412553298172,-0.0551726700606049,
-0.333589372248002));
#37267=CARTESIAN_POINT('Ctrl Pts',(0.141425907488028,0.117525742149486,
-0.322469726506402));
#37268=CARTESIAN_POINT('Ctrl Pts',(-0.0221344224967506,0.182547677935732,
-0.311350080764802));
#37269=CARTESIAN_POINT('Ctrl Pts',(-0.165415309183955,0.0803203763697784,
-0.300230435023202));
#37270=CARTESIAN_POINT('Ctrl Pts',(-0.157143546107041,-0.0954960381063839,
-0.289110789281602));
#37271=CARTESIAN_POINT('Ctrl Pts',(-0.00489767969399011,-0.183819477000074,
-0.277991143540001));
#37272=CARTESIAN_POINT('Ctrl Pts',(0.151835415403586,-0.103728462705588,
-0.266871497798402));
#37273=CARTESIAN_POINT('Ctrl Pts',(0.169457689254605,0.0713980317726476,
-0.255751852056801));
#37274=CARTESIAN_POINT('Ctrl Pts',(0.0318237052925425,0.181110019726059,
-0.244632206315202));
#37275=CARTESIAN_POINT('Ctrl Pts',(-0.134966992047393,0.12488994440001,
-0.233512560573601));
#37276=CARTESIAN_POINT('Ctrl Pts',(-0.178101631312305,-0.0457536495135279,
-0.222392914832001));
#37277=CARTESIAN_POINT('Ctrl Pts',(-0.0580604758392629,-0.174477990107862,
-0.211273269090402));
#37278=CARTESIAN_POINT('Ctrl Pts',(0.115175382590983,-0.143346492982138,
-0.200153623348801));
#37279=CARTESIAN_POINT('Ctrl Pts',(0.182888160188203,0.0191183062440436,
-0.189033977607201));
#37280=CARTESIAN_POINT('Ctrl Pts',(0.0830397364904521,0.164067036179902,
-0.177914331865601));
#37281=CARTESIAN_POINT('Ctrl Pts',(-0.0928892335709049,0.158698351565871,
-0.166794686124001));
#37282=CARTESIAN_POINT('Ctrl Pts',(-0.183713626385541,0.00793114559592943,
-0.155675040382401));
#37283=CARTESIAN_POINT('Ctrl Pts',(-0.106220436282912,-0.150102699871419,
-0.144555394640801));
#37284=CARTESIAN_POINT('Ctrl Pts',(0.0685911587771073,-0.170612914816246,
-0.133435748899201));
#37285=CARTESIAN_POINT('Ctrl Pts',(0.180560286830463,-0.0348090586500559,
-0.122316103157601));
#37286=CARTESIAN_POINT('Ctrl Pts',(0.127100258123179,0.132887815499814,
-0.111196457416001));
#37287=CARTESIAN_POINT('Ctrl Pts',(-0.0428069278985511,0.17883139309898,
-0.100076811674401));
#37288=CARTESIAN_POINT('Ctrl Pts',(-0.173497372046971,0.0609347022767939,
-0.0889571659328004));
#37289=CARTESIAN_POINT('Ctrl Pts',(-0.145225197994402,-0.112797907004394,
-0.0778375201912004));
#37290=CARTESIAN_POINT('Ctrl Pts',(0.0160916033347015,-0.183170692569655,
-0.0667178744496004));
#37291=CARTESIAN_POINT('Ctrl Pts',(0.16268430194739,-0.0857519355616629,
-0.0555982287080002));
#37292=CARTESIAN_POINT('Ctrl Pts',(0.160190409020898,0.0902865901057441,
-0.0444785829664002));
#37293=CARTESIAN_POINT('Ctrl Pts',(0.0109996935541243,0.183501383580361,
-0.0333589372248001));
#37294=CARTESIAN_POINT('Ctrl Pts',(-0.148400842830771,0.108792702151384,
-0.0222392914832001));
#37295=CARTESIAN_POINT('Ctrl Pts',(-0.171577704761274,-0.0659904817000804,
-0.0111196457416));
#37296=CARTESIAN_POINT('Ctrl Pts',(-0.0826091653404253,-0.141597064818995,
-0.00370654858053334));
#37297=CARTESIAN_POINT('Ctrl Pts',(-0.0319621170202048,-0.15223082991164,
0.));
#37298=CARTESIAN_POINT('Ctrl Pts',(0.134904440327165,0.101515941725715,
-1.01533827215147));
#37299=CARTESIAN_POINT('Ctrl Pts',(0.101130185737347,0.146398517166105,
-1.01163172357094));
#37300=CARTESIAN_POINT('Ctrl Pts',(-0.0141505916566728,0.199026458780906,
-1.00421862640987));
#37301=CARTESIAN_POINT('Ctrl Pts',(-0.175266576578065,0.0957600367360653,
-0.99309898066827));
#37302=CARTESIAN_POINT('Ctrl Pts',(-0.175292338522647,-0.0953125528950821,
-0.981979334926671));
#37303=CARTESIAN_POINT('Ctrl Pts',(-0.0149730577468432,-0.199022465345967,
-0.970859689185071));
#37304=CARTESIAN_POINT('Ctrl Pts',(0.159197993862087,-0.120408928537827,
-0.95974004344347));
#37305=CARTESIAN_POINT('Ctrl Pts',(0.18744269558271,0.0685331036176038,
-0.94862039770187));
#37306=CARTESIAN_POINT('Ctrl Pts',(0.043990101659657,0.194679967594623,
-0.937500751960271));
#37307=CARTESIAN_POINT('Ctrl Pts',(-0.139785285225796,0.142464938577181,
-0.92638110621867));
#37308=CARTESIAN_POINT('Ctrl Pts',(-0.195479986736384,-0.0402772449093781,
-0.915261460477071));
#37309=CARTESIAN_POINT('Ctrl Pts',(-0.0720822573311022,-0.186116829254826,
-0.90414181473547));
#37310=CARTESIAN_POINT('Ctrl Pts',(0.117359657534594,-0.161437556325261,
-0.89302216899387));
#37311=CARTESIAN_POINT('Ctrl Pts',(0.19927579412211,0.0111501893662626,
-0.88190252325227));
#37312=CARTESIAN_POINT('Ctrl Pts',(0.098617250796205,0.173522073986237,
-0.87078287751067));
#37313=CARTESIAN_POINT('Ctrl Pts',(-0.092394311950167,0.176913993440523,
-0.859663231769071));
#37314=CARTESIAN_POINT('Ctrl Pts',(-0.198754471849409,0.0182181963201783,
-0.848543586027468));
#37315=CARTESIAN_POINT('Ctrl Pts',(-0.123016925426643,-0.157169001233487,
-0.837423940285871));
#37316=CARTESIAN_POINT('Ctrl Pts',(0.0654281497715049,-0.188558782418071,
-0.826304294544269));
#37317=CARTESIAN_POINT('Ctrl Pts',(0.193928262115897,-0.0471919788599082,
-0.815184648802669));
#37318=CARTESIAN_POINT('Ctrl Pts',(0.144752321008073,0.137411868959591,
-0.80406500306107));
#37319=CARTESIAN_POINT('Ctrl Pts',(-0.0370449556086742,0.196119675198496,
-0.792945357319469));
#37320=CARTESIAN_POINT('Ctrl Pts',(-0.184901831244498,0.0751436498183813,
-0.781825711577869));
#37321=CARTESIAN_POINT('Ctrl Pts',(-0.163352608820018,-0.114678598097066,
-0.770706065836269));
#37322=CARTESIAN_POINT('Ctrl Pts',(0.00785942923184284,-0.199432908401222,
-0.75958642009467));
#37323=CARTESIAN_POINT('Ctrl Pts',(0.17187069826933,-0.101467820552112,
-0.748466774353069));
#37324=CARTESIAN_POINT('Ctrl Pts',(0.178414923801518,0.0894615590575204,
-0.737347128611469));
#37325=CARTESIAN_POINT('Ctrl Pts',(0.0214963197624508,0.19842672149802,
-0.726227482869868));
#37326=CARTESIAN_POINT('Ctrl Pts',(-0.155117101045983,0.125594349098855,
-0.71510783712827));
#37327=CARTESIAN_POINT('Ctrl Pts',(-0.189613037088232,-0.0623069156368273,
-0.703988191386669));
#37328=CARTESIAN_POINT('Ctrl Pts',(-0.0503864902998775,-0.193122906881706,
-0.692868545645069));
#37329=CARTESIAN_POINT('Ctrl Pts',(0.135003897997258,-0.147000690788359,
-0.681748899903469));
#37330=CARTESIAN_POINT('Ctrl Pts',(0.196704413977544,0.0338027970662945,
-0.670629254161869));
#37331=CARTESIAN_POINT('Ctrl Pts',(0.0781853643609582,0.183636337272974,
-0.659509608420269));
#37332=CARTESIAN_POINT('Ctrl Pts',(-0.111966711254192,0.16522321609927,
-0.648389962678668));
#37333=CARTESIAN_POINT('Ctrl Pts',(-0.199535465758804,-0.0045665601741977,
-0.637270316937069));
#37334=CARTESIAN_POINT('Ctrl Pts',(-0.10429085968633,-0.170172477660811,
-0.626150671195469));
#37335=CARTESIAN_POINT('Ctrl Pts',(0.086504492034861,-0.179867252230991,
-0.615031025453868));
#37336=CARTESIAN_POINT('Ctrl Pts',(0.198044876055494,-0.0247685816210578,
-0.603911379712269));
#37337=CARTESIAN_POINT('Ctrl Pts',(0.128137570067725,0.153022935223718,
-0.592791733970668));
#37338=CARTESIAN_POINT('Ctrl Pts',(-0.0591687141473076,0.190615631136323,
-0.581672088229069));
#37339=CARTESIAN_POINT('Ctrl Pts',(-0.192264928823459,0.0535672727685228,
-0.570552442487468));
#37340=CARTESIAN_POINT('Ctrl Pts',(-0.149209011217944,-0.132559143549997,
-0.559432796745868));
#37341=CARTESIAN_POINT('Ctrl Pts',(0.0305514298933165,-0.197235558910708,
-0.548313151004268));
#37342=CARTESIAN_POINT('Ctrl Pts',(0.182320809125048,-0.0812057764406795,
-0.537193505262669));
#37343=CARTESIAN_POINT('Ctrl Pts',(0.167048807054298,0.109224317938277,
-0.526073859521067));
#37344=CARTESIAN_POINT('Ctrl Pts',(-0.00127244709684963,0.199583657762181,
-0.514954213779468));
#37345=CARTESIAN_POINT('Ctrl Pts',(-0.168427891806321,0.107085483745576,
-0.503834568037868));
#37346=CARTESIAN_POINT('Ctrl Pts',(-0.181270574126195,-0.083523856013151,
-0.492714922296267));
#37347=CARTESIAN_POINT('Ctrl Pts',(-0.0280340950116467,-0.197609071361169,
-0.481595276554668));
#37348=CARTESIAN_POINT('Ctrl Pts',(0.150887076798065,-0.130645878705303,
-0.470475630813067));
#37349=CARTESIAN_POINT('Ctrl Pts',(0.19156629010618,0.0560143915641372,
-0.459355985071468));
#37350=CARTESIAN_POINT('Ctrl Pts',(0.056733460308012,0.191354566312969,
-0.448236339329867));
#37351=CARTESIAN_POINT('Ctrl Pts',(-0.130078272070719,0.151376678198602,
-0.437116693588267));
#37352=CARTESIAN_POINT('Ctrl Pts',(-0.197712965095534,-0.0272917386854921,
-0.425997047846668));
#37353=CARTESIAN_POINT('Ctrl Pts',(-0.0842040632149887,-0.180955605896666,
-0.414877402105067));
#37354=CARTESIAN_POINT('Ctrl Pts',(0.106452165392644,-0.168828883934509,
-0.403757756363467));
#37355=CARTESIAN_POINT('Ctrl Pts',(0.199577471253882,-0.00202201267109366,
-0.392638110621867));
#37356=CARTESIAN_POINT('Ctrl Pts',(0.109850931321565,0.166637416131906,
-0.381518464880267));
#37357=CARTESIAN_POINT('Ctrl Pts',(-0.0805204631032623,0.182624507087749,
-0.370398819138667));
#37358=CARTESIAN_POINT('Ctrl Pts',(-0.197119426150196,0.0312919702397112,
-0.359279173397067));
#37359=CARTESIAN_POINT('Ctrl Pts',(-0.133118591600838,-0.148710107717997,
-0.348159527655467));
#37360=CARTESIAN_POINT('Ctrl Pts',(0.0528448073149077,-0.192464754975046,
-0.337039881913867));
#37361=CARTESIAN_POINT('Ctrl Pts',(0.190392067385672,-0.05988419026186,
-0.325920236172266));
#37362=CARTESIAN_POINT('Ctrl Pts',(0.153503101130798,0.127561959495798,
-0.314800590430667));
#37363=CARTESIAN_POINT('Ctrl Pts',(-0.024024611581707,0.198136502463191,
-0.303680944689066));
#37364=CARTESIAN_POINT('Ctrl Pts',(-0.179541099542854,0.0871794077601917,
-0.292561298947467));
#37365=CARTESIAN_POINT('Ctrl Pts',(-0.170562961755526,-0.103651008895067,
-0.281441653205866));
#37366=CARTESIAN_POINT('Ctrl Pts',(-0.00531592149363913,-0.19951690796215,
-0.270322007464267));
#37367=CARTESIAN_POINT('Ctrl Pts',(0.164801538416192,-0.112586448859704,
-0.259202361722666));
#37368=CARTESIAN_POINT('Ctrl Pts',(0.183928682326064,0.0774951314536493,
-0.248082715981066));
#37369=CARTESIAN_POINT('Ctrl Pts',(0.0345413194699957,0.196576074126752,
-0.236963070239466));
#37370=CARTESIAN_POINT('Ctrl Pts',(-0.146492620747893,0.135555034476814,
-0.225843424497866));
#37371=CARTESIAN_POINT('Ctrl Pts',(-0.193310781655808,-0.0496608239121424,
-0.214723778756266));
#37372=CARTESIAN_POINT('Ctrl Pts',(-0.0630186028342171,-0.18937769632408,
-0.203604133014666));
#37373=CARTESIAN_POINT('Ctrl Pts',(0.125010888851029,-0.155587696765142,
-0.192484487273065));
#37374=CARTESIAN_POINT('Ctrl Pts',(0.198506060506429,0.0207509313459927,
-0.181364841531466));
#37375=CARTESIAN_POINT('Ctrl Pts',(0.0901309901048207,0.178077689542741,
-0.170245195789865));
#37376=CARTESIAN_POINT('Ctrl Pts',(-0.100821593921917,0.172250541236717,
-0.159125550048266));
#37377=CARTESIAN_POINT('Ctrl Pts',(-0.199402018138383,0.00860843296761797,
-0.148005904306665));
#37378=CARTESIAN_POINT('Ctrl Pts',(-0.115291226780875,-0.162920856069588,
-0.136886258565066));
#37379=CARTESIAN_POINT('Ctrl Pts',(0.0744485629928304,-0.185182559422327,
-0.125766612823465));
#37380=CARTESIAN_POINT('Ctrl Pts',(0.195979396291931,-0.0377816097851794,
-0.114646967081865));
#37381=CARTESIAN_POINT('Ctrl Pts',(0.137954099945121,0.144235891033227,
-0.103527321340265));
#37382=CARTESIAN_POINT('Ctrl Pts',(-0.046462464332188,0.194102862112147,
-0.092407675598665));
#37383=CARTESIAN_POINT('Ctrl Pts',(-0.188313337494461,0.0661382764452947,
-0.0812880298570651));
#37384=CARTESIAN_POINT('Ctrl Pts',(-0.157626835495907,-0.12243038658036,
-0.0701683841154649));
#37385=CARTESIAN_POINT('Ctrl Pts',(0.0174657603964976,-0.19881271999685,
-0.0590487383738649));
#37386=CARTESIAN_POINT('Ctrl Pts',(0.176576875466308,-0.093074799875673,
-0.0479290926322647));
#37387=CARTESIAN_POINT('Ctrl Pts',(0.173870014291407,0.0979966953574602,
-0.0368094468906647));
#37388=CARTESIAN_POINT('Ctrl Pts',(0.0119390223618658,0.199171650666351,
-0.0256898011490646));
#37389=CARTESIAN_POINT('Ctrl Pts',(-0.161073667403376,0.118083153626222,
-0.0145701554074646));
#37390=CARTESIAN_POINT('Ctrl Pts',(-0.186229738479772,-0.0716257987380052,
-0.00345050966586453));
#37391=CARTESIAN_POINT('Ctrl Pts',(-0.0896636499409105,-0.15368887459728,
0.00396258749520215));
#37392=CARTESIAN_POINT('Ctrl Pts',(-0.0346915509926802,-0.165230719704802,
0.00766913607573549));
#37393=CARTESIAN_POINT('Ctrl Pts',(0.145518343480251,0.10950293141529,-1.00766913607574));
#37394=CARTESIAN_POINT('Ctrl Pts',(0.109086825227246,0.157916742060614,
-1.0039625874952));
#37395=CARTESIAN_POINT('Ctrl Pts',(-0.0152639205362734,0.214685302576403,
-0.996549490334137));
#37396=CARTESIAN_POINT('Ctrl Pts',(-0.18905605945395,0.103294167958045,
-0.985429844592534));
#37397=CARTESIAN_POINT('Ctrl Pts',(-0.189083848276107,-0.102811477342996,
-0.974310198850937));
#37398=CARTESIAN_POINT('Ctrl Pts',(-0.0161510959525931,-0.214680994949199,
-0.963190553109335));
#37399=CARTESIAN_POINT('Ctrl Pts',(0.171723245699015,-0.129882365462275,
-0.952070907367735));
#37400=CARTESIAN_POINT('Ctrl Pts',(0.202190161365477,0.0739250960739926,
-0.940951261626135));
#37401=CARTESIAN_POINT('Ctrl Pts',(0.0474511195296233,0.209996841649205,
-0.929831615884535));
#37402=CARTESIAN_POINT('Ctrl Pts',(-0.150783199571793,0.153673680536314,
-0.918711970142935));
#37403=CARTESIAN_POINT('Ctrl Pts',(-0.210859804054144,-0.0434461456194237,
-0.907592324401335));
#37404=CARTESIAN_POINT('Ctrl Pts',(-0.0777534872514279,-0.200759979592051,
-0.896472678659735));
#37405=CARTESIAN_POINT('Ctrl Pts',(0.126593186365301,-0.174139010658059,
-0.885353032918134));
#37406=CARTESIAN_POINT('Ctrl Pts',(0.214954254923228,0.0120274550054429,
-0.874233387176536));
#37407=CARTESIAN_POINT('Ctrl Pts',(0.106376179610083,0.187174304289003,
-0.863113741434934));
#37408=CARTESIAN_POINT('Ctrl Pts',(-0.0996636373819806,0.190833090456525,
-0.851994095693334));
#37409=CARTESIAN_POINT('Ctrl Pts',(-0.214391916475665,0.0196515529309577,
-0.840874449951735));
#37410=CARTESIAN_POINT('Ctrl Pts',(-0.132695552234643,-0.169534617618786,
-0.829754804210134));
#37411=CARTESIAN_POINT('Ctrl Pts',(0.0705758531641878,-0.203394058784034,
-0.818635158468534));
#37412=CARTESIAN_POINT('Ctrl Pts',(0.209185994090859,-0.0509049114513555,
-0.807515512726934));
#37413=CARTESIAN_POINT('Ctrl Pts',(0.15614102780407,0.148223049567763,-0.796395866985335));
#37414=CARTESIAN_POINT('Ctrl Pts',(-0.0399595488584374,0.211549821411053,
-0.785276221243734));
#37415=CARTESIAN_POINT('Ctrl Pts',(-0.199449388944583,0.0810557415168278,
-0.774156575502134));
#37416=CARTESIAN_POINT('Ctrl Pts',(-0.176204734114151,-0.123701188687723,
-0.763036929760533));
#37417=CARTESIAN_POINT('Ctrl Pts',(0.00847778708947041,-0.215123730513342,
-0.751917284018934));
#37418=CARTESIAN_POINT('Ctrl Pts',(0.185393002960411,-0.109451024202659,
-0.740797638277333));
#37419=CARTESIAN_POINT('Ctrl Pts',(0.192452109810384,0.0965001437138712,
-0.729677992535734));
#37420=CARTESIAN_POINT('Ctrl Pts',(0.0231875899352727,0.214038379645495,
-0.718558346794133));
#37421=CARTESIAN_POINT('Ctrl Pts',(-0.167321279677142,0.135475760375439,
-0.707438701052534));
#37422=CARTESIAN_POINT('Ctrl Pts',(-0.204531259255984,-0.0672090490783415,
-0.696319055310933));
#37423=CARTESIAN_POINT('Ctrl Pts',(-0.0543507580954369,-0.208317275764699,
-0.685199409569334));
#37424=CARTESIAN_POINT('Ctrl Pts',(0.14562562620099,-0.158566293015243,
-0.674079763827733));
#37425=CARTESIAN_POINT('Ctrl Pts',(0.21218056579789,0.0364623063715093,
-0.662960118086133));
#37426=CARTESIAN_POINT('Ctrl Pts',(0.0843367696320044,0.198084329455259,
-0.651840472344534));
#37427=CARTESIAN_POINT('Ctrl Pts',(-0.120775938190972,0.178222515529785,
-0.640720826602933));
#37428=CARTESIAN_POINT('Ctrl Pts',(-0.215234356796293,-0.00492584432610516,
-0.629601180861333));
#37429=CARTESIAN_POINT('Ctrl Pts',(-0.112496172141415,-0.183561171115467,
-0.618481535119733));
#37430=CARTESIAN_POINT('Ctrl Pts',(0.0933104229481655,-0.194018703369007,
-0.607361889378134));
#37431=CARTESIAN_POINT('Ctrl Pts',(0.213626491674075,-0.0267173041829527,
-0.596242243636532));
#37432=CARTESIAN_POINT('Ctrl Pts',(0.138219074840083,0.165062350759088,
-0.585122597894933));
#37433=CARTESIAN_POINT('Ctrl Pts',(-0.0638239426937432,0.205612734592953,
-0.574002952153332));
#37434=CARTESIAN_POINT('Ctrl Pts',(-0.207391794398217,0.0577817956112202,
-0.562883306411733));
#37435=CARTESIAN_POINT('Ctrl Pts',(-0.160948357905082,-0.14298852532782,
-0.551763660670132));
#37436=CARTESIAN_POINT('Ctrl Pts',(0.032955130744744,-0.212753499725302,
-0.540644014928533));
#37437=CARTESIAN_POINT('Ctrl Pts',(0.196665299240809,-0.0875948192662701,
-0.529524369186932));
#37438=CARTESIAN_POINT('Ctrl Pts',(0.180191738863013,0.117817781057408,
-0.518404723445332));
#37439=CARTESIAN_POINT('Ctrl Pts',(-0.00137255966705475,0.215286340411388,
-0.507285077703732));
#37440=CARTESIAN_POINT('Ctrl Pts',(-0.181679326136985,0.115510669386764,
-0.496165431962132));
#37441=CARTESIAN_POINT('Ctrl Pts',(-0.195532434696637,-0.0900952788406405,
-0.485045786220532));
#37442=CARTESIAN_POINT('Ctrl Pts',(-0.0302397390120705,-0.213156399088203,
-0.473926140478932));
#37443=CARTESIAN_POINT('Ctrl Pts',(0.162758448980498,-0.140924730169087,
-0.462806494737332));
#37444=CARTESIAN_POINT('Ctrl Pts',(0.206638188745334,0.060421446853042,
-0.451686848995732));
#37445=CARTESIAN_POINT('Ctrl Pts',(0.0611970899097395,0.206409807117652,
-0.440567203254132));
#37446=CARTESIAN_POINT('Ctrl Pts',(-0.140312465835808,0.163286570846607,
-0.429447557512532));
#37447=CARTESIAN_POINT('Ctrl Pts',(-0.213268466890316,-0.0294389761714076,
-0.418327911770931));
#37448=CARTESIAN_POINT('Ctrl Pts',(-0.0908290028381239,-0.195192685649839,
-0.407208266029332));
#37449=CARTESIAN_POINT('Ctrl Pts',(0.114827523321364,-0.182111867201617,
-0.396088620287731));
#37450=CARTESIAN_POINT('Ctrl Pts',(0.215279667165959,-0.0021810989592354,
-0.384968974546132));
#37451=CARTESIAN_POINT('Ctrl Pts',(0.118493694624951,0.179747980856202,
-0.373849328804531));
#37452=CARTESIAN_POINT('Ctrl Pts',(-0.0868555873967757,0.196992891307782,
-0.362729683062932));
#37453=CARTESIAN_POINT('Ctrl Pts',(-0.212628229964777,0.0337539347294509,
-0.351610037321331));
#37454=CARTESIAN_POINT('Ctrl Pts',(-0.14359198918286,-0.160410202076461,
-0.340490391579732));
#37455=CARTESIAN_POINT('Ctrl Pts',(0.0570024886011833,-0.207607342311188,
-0.329370745838131));
#37456=CARTESIAN_POINT('Ctrl Pts',(0.205371581473172,-0.0645957104631151,
-0.318251100096531));
#37457=CARTESIAN_POINT('Ctrl Pts',(0.165580294773567,0.13759817684211,-0.307131454354931));
#37458=CARTESIAN_POINT('Ctrl Pts',(-0.0259148006666635,0.213725326990651,
-0.296011808613331));
#37459=CARTESIAN_POINT('Ctrl Pts',(-0.193666889901754,0.0940384391506045,
-0.284892162871731));
#37460=CARTESIAN_POINT('Ctrl Pts',(-0.183982377404012,-0.11180597968375,
-0.27377251713013));
#37461=CARTESIAN_POINT('Ctrl Pts',(-0.00573416329328779,-0.215214338924227,
-0.262652871388531));
#37462=CARTESIAN_POINT('Ctrl Pts',(0.177767661428798,-0.12144443501382,
-0.25153322564693));
#37463=CARTESIAN_POINT('Ctrl Pts',(0.198399675397523,0.0835922311346511,
-0.240413579905331));
#37464=CARTESIAN_POINT('Ctrl Pts',(0.0372589336474485,0.212042128527444,
-0.22929393416373));
#37465=CARTESIAN_POINT('Ctrl Pts',(-0.158018249448392,0.146220124553619,
-0.218174288422131));
#37466=CARTESIAN_POINT('Ctrl Pts',(-0.20851993199931,-0.0535679983107572,
-0.20705464268053));
#37467=CARTESIAN_POINT('Ctrl Pts',(-0.0679767298291708,-0.204277402540297,
-0.195934996938931));
#37468=CARTESIAN_POINT('Ctrl Pts',(0.134846395111074,-0.167828900548145,
-0.18481535119733));
#37469=CARTESIAN_POINT('Ctrl Pts',(0.214123960824655,0.0223835564479417,
-0.17369570545573));
#37470=CARTESIAN_POINT('Ctrl Pts',(0.097222243719189,0.19208834290558,-0.16257605971413));
#37471=CARTESIAN_POINT('Ctrl Pts',(-0.10875395427293,0.185802730907562,
-0.15145641397253));
#37472=CARTESIAN_POINT('Ctrl Pts',(-0.215090409891226,0.0092857203393065,
-0.14033676823093));
#37473=CARTESIAN_POINT('Ctrl Pts',(-0.124362017278838,-0.175739012267757,
-0.12921712248933));
#37474=CARTESIAN_POINT('Ctrl Pts',(0.0803059672085533,-0.199752204028408,
-0.11809747674773));
#37475=CARTESIAN_POINT('Ctrl Pts',(0.211398505753398,-0.0407541609203029,
-0.10697783100613));
#37476=CARTESIAN_POINT('Ctrl Pts',(0.148807941767063,0.15558396656664,-0.0958581852645297));
#37477=CARTESIAN_POINT('Ctrl Pts',(-0.0501180007658248,0.209374331125314,
-0.0847385395229296));
#37478=CARTESIAN_POINT('Ctrl Pts',(-0.203129302941952,0.0713418506137954,
-0.0736188937813295));
#37479=CARTESIAN_POINT('Ctrl Pts',(-0.170028472997412,-0.132062866156327,
-0.0624992480397294));
#37480=CARTESIAN_POINT('Ctrl Pts',(0.018839917458294,-0.214454747424046,
-0.0513796022981294));
#37481=CARTESIAN_POINT('Ctrl Pts',(0.190469448985226,-0.100397664189683,
-0.0402599565565293));
#37482=CARTESIAN_POINT('Ctrl Pts',(0.187549619561917,0.105706800609176,
-0.0291403108149292));
#37483=CARTESIAN_POINT('Ctrl Pts',(0.0128783511696067,0.214841917752341,
-0.0180206650733292));
#37484=CARTESIAN_POINT('Ctrl Pts',(-0.17374649197598,0.12737360510106,-0.00690101933172906));
#37485=CARTESIAN_POINT('Ctrl Pts',(-0.20088177219827,-0.07726111577593,
0.00421862640987097));
#37486=CARTESIAN_POINT('Ctrl Pts',(-0.0967181345413958,-0.165780684375565,
0.0116317235709377));
#37487=CARTESIAN_POINT('Ctrl Pts',(-0.0374209849651557,-0.178230609497963,
0.015338272151471));
#37488=CARTESIAN_POINT('Ctrl Pts',(0.156132246633336,0.117489921104864,
-1.));
#37489=CARTESIAN_POINT('Ctrl Pts',(0.117043464717144,0.169434966955123,
-0.996293451419467));
#37490=CARTESIAN_POINT('Ctrl Pts',(-0.0163772494158741,0.2303441463719,
-0.9888803542584));
#37491=CARTESIAN_POINT('Ctrl Pts',(-0.202845542329835,0.110828299180025,
-0.9777607085168));
#37492=CARTESIAN_POINT('Ctrl Pts',(-0.202875358029568,-0.11031040179091,
-0.9666410627752));
#37493=CARTESIAN_POINT('Ctrl Pts',(-0.0173291341583431,-0.23033952455243,
-0.9555214170336));
#37494=CARTESIAN_POINT('Ctrl Pts',(0.184248497535942,-0.139355802386723,
-0.944401771292));
#37495=CARTESIAN_POINT('Ctrl Pts',(0.216937627148243,0.0793170885303813,
-0.933282125550399));
#37496=CARTESIAN_POINT('Ctrl Pts',(0.0509121373995896,0.225313715703786,
-0.922162479808799));
#37497=CARTESIAN_POINT('Ctrl Pts',(-0.161781113917791,0.164882422495448,
-0.9110428340672));
#37498=CARTESIAN_POINT('Ctrl Pts',(-0.226239621371903,-0.0466150463294693,
-0.899923188325598));
#37499=CARTESIAN_POINT('Ctrl Pts',(-0.0834247171717535,-0.215403129929277,
-0.888803542584));
#37500=CARTESIAN_POINT('Ctrl Pts',(0.135826715196008,-0.186840464990857,
-0.877683896842398));
#37501=CARTESIAN_POINT('Ctrl Pts',(0.230632715724346,0.0129047206446236,
-0.866564251100799));
#37502=CARTESIAN_POINT('Ctrl Pts',(0.114135108423961,0.200826534591769,
-0.855444605359199));
#37503=CARTESIAN_POINT('Ctrl Pts',(-0.106932962813794,0.204752187472527,
-0.8443249596176));
#37504=CARTESIAN_POINT('Ctrl Pts',(-0.230029361101922,0.0210849095417369,
-0.833205313875998));
#37505=CARTESIAN_POINT('Ctrl Pts',(-0.142374179042644,-0.181900234004086,
-0.8220856681344));
#37506=CARTESIAN_POINT('Ctrl Pts',(0.0757235565568705,-0.218229335149998,
-0.810966022392799));
#37507=CARTESIAN_POINT('Ctrl Pts',(0.224443726065821,-0.0546178440428023,
-0.799846376651198));
#37508=CARTESIAN_POINT('Ctrl Pts',(0.167529734600066,0.159034230175935,
-0.788726730909599));
#37509=CARTESIAN_POINT('Ctrl Pts',(-0.0428741421082007,0.22697996762361,
-0.777607085167998));
#37510=CARTESIAN_POINT('Ctrl Pts',(-0.213996946644668,0.0869678332152738,
-0.766487439426399));
#37511=CARTESIAN_POINT('Ctrl Pts',(-0.189056859408284,-0.132723779278379,
-0.755367793684799));
#37512=CARTESIAN_POINT('Ctrl Pts',(0.00909614494709787,-0.230814552625462,
-0.744248147943198));
#37513=CARTESIAN_POINT('Ctrl Pts',(0.198915307651492,-0.117434227853206,
-0.733128502201599));
#37514=CARTESIAN_POINT('Ctrl Pts',(0.20648929581925,0.103538728370222,-0.722008856459998));
#37515=CARTESIAN_POINT('Ctrl Pts',(0.0248788601080945,0.22965003779297,
-0.710889210718398));
#37516=CARTESIAN_POINT('Ctrl Pts',(-0.179525458308301,0.145357171652024,
-0.699769564976799));
#37517=CARTESIAN_POINT('Ctrl Pts',(-0.219449481423736,-0.0721111825198558,
-0.688649919235197));
#37518=CARTESIAN_POINT('Ctrl Pts',(-0.0583150258909959,-0.223511644647691,
-0.677530273493599));
#37519=CARTESIAN_POINT('Ctrl Pts',(0.156247354404722,-0.170131895242127,
-0.666410627751997));
#37520=CARTESIAN_POINT('Ctrl Pts',(0.227656717618236,0.0391218156767241,
-0.655290982010398));
#37521=CARTESIAN_POINT('Ctrl Pts',(0.0904881749030501,0.212532321637545,
-0.644171336268797));
#37522=CARTESIAN_POINT('Ctrl Pts',(-0.129585165127752,0.191221814960301,
-0.633051690527198));
#37523=CARTESIAN_POINT('Ctrl Pts',(-0.230933247833782,-0.00528512847801286,
-0.621932044785597));
#37524=CARTESIAN_POINT('Ctrl Pts',(-0.120701484596501,-0.196949864570122,
-0.610812399043998));
#37525=CARTESIAN_POINT('Ctrl Pts',(0.10011635386147,-0.208170154507023,
-0.599692753302397));
#37526=CARTESIAN_POINT('Ctrl Pts',(0.229208107292656,-0.0286660267448476,
-0.588573107560798));
#37527=CARTESIAN_POINT('Ctrl Pts',(0.148300579612441,0.177101766294457,
-0.577453461819196));
#37528=CARTESIAN_POINT('Ctrl Pts',(-0.0684791712401787,0.220609838049582,
-0.566333816077598));
#37529=CARTESIAN_POINT('Ctrl Pts',(-0.222518659972974,0.0619963184539177,
-0.555214170335996));
#37530=CARTESIAN_POINT('Ctrl Pts',(-0.17268770459222,-0.153417907105642,
-0.544094524594398));
#37531=CARTESIAN_POINT('Ctrl Pts',(0.0353588315961715,-0.228271440539896,
-0.532974878852797));
#37532=CARTESIAN_POINT('Ctrl Pts',(0.21100978935657,-0.0939838620918607,
-0.521855233111197));
#37533=CARTESIAN_POINT('Ctrl Pts',(0.193334670671728,0.126411244176538,
-0.510735587369597));
#37534=CARTESIAN_POINT('Ctrl Pts',(-0.00147267223725966,0.230989023060594,
-0.499615941627997));
#37535=CARTESIAN_POINT('Ctrl Pts',(-0.19493076046765,0.123935855027952,
-0.488496295886396));
#37536=CARTESIAN_POINT('Ctrl Pts',(-0.20979429526708,-0.0966667016681302,
-0.477376650144797));
#37537=CARTESIAN_POINT('Ctrl Pts',(-0.0324453830124945,-0.228703726815237,
-0.466257004403196));
#37538=CARTESIAN_POINT('Ctrl Pts',(0.174629821162932,-0.151203581632872,
-0.455137358661597));
#37539=CARTESIAN_POINT('Ctrl Pts',(0.221710087384488,0.0648285021419467,
-0.444017712919996));
#37540=CARTESIAN_POINT('Ctrl Pts',(0.0656607195114666,0.221465047922334,
-0.432898067178396));
#37541=CARTESIAN_POINT('Ctrl Pts',(-0.150546659600897,0.175196463494612,
-0.421778421436796));
#37542=CARTESIAN_POINT('Ctrl Pts',(-0.228823968685098,-0.0315862136573233,
-0.410658775695196));
#37543=CARTESIAN_POINT('Ctrl Pts',(-0.0974539424612588,-0.209429765403011,
-0.399539129953596));
#37544=CARTESIAN_POINT('Ctrl Pts',(0.123202881250083,-0.195394850468726,
-0.388419484211996));
#37545=CARTESIAN_POINT('Ctrl Pts',(0.230981863078037,-0.00234018524737671,
-0.377299838470396));
#37546=CARTESIAN_POINT('Ctrl Pts',(0.127136457928336,0.192858545580498,
-0.366180192728797));
#37547=CARTESIAN_POINT('Ctrl Pts',(-0.0931907116902888,0.211361275527816,
-0.355060546987195));
#37548=CARTESIAN_POINT('Ctrl Pts',(-0.228137033779358,0.0362158992191905,
-0.343940901245597));
#37549=CARTESIAN_POINT('Ctrl Pts',(-0.154065386764881,-0.172110296434925,
-0.332821255503995));
#37550=CARTESIAN_POINT('Ctrl Pts',(0.0611601698874586,-0.22274992964733,
-0.321701609762396));
#37551=CARTESIAN_POINT('Ctrl Pts',(0.220351095560672,-0.0693072306643703,
-0.310581964020795));
#37552=CARTESIAN_POINT('Ctrl Pts',(0.177657488416336,0.147634394188423,
-0.299462318279196));
#37553=CARTESIAN_POINT('Ctrl Pts',(-0.0278049897516198,0.22931415151811,
-0.288342672537595));
#37554=CARTESIAN_POINT('Ctrl Pts',(-0.207792680260653,0.100897470541018,
-0.277223026795995));
#37555=CARTESIAN_POINT('Ctrl Pts',(-0.197401793052498,-0.119960950472433,
-0.266103381054396));
#37556=CARTESIAN_POINT('Ctrl Pts',(-0.00615240509293671,-0.230911769886303,
-0.254983735312795));
#37557=CARTESIAN_POINT('Ctrl Pts',(0.190733784441404,-0.130302421167936,
-0.243864089571195));
#37558=CARTESIAN_POINT('Ctrl Pts',(0.212870668468982,0.0896893308156527,
-0.232744443829595));
#37559=CARTESIAN_POINT('Ctrl Pts',(0.0399765478249015,0.227508182928137,
-0.221624798087995));
#37560=CARTESIAN_POINT('Ctrl Pts',(-0.169543878148892,0.156885214630423,
-0.210505152346395));
#37561=CARTESIAN_POINT('Ctrl Pts',(-0.223729082342813,-0.0574751727093715,
-0.199385506604795));
#37562=CARTESIAN_POINT('Ctrl Pts',(-0.0729348568241247,-0.219177108756516,
-0.188265860863195));
#37563=CARTESIAN_POINT('Ctrl Pts',(0.144681901371119,-0.180070104331149,
-0.177146215121594));
#37564=CARTESIAN_POINT('Ctrl Pts',(0.22974186114288,0.0240161815498906,
-0.166026569379995));
#37565=CARTESIAN_POINT('Ctrl Pts',(0.104313497333558,0.206098996268419,
-0.154906923638395));
#37566=CARTESIAN_POINT('Ctrl Pts',(-0.116686314623943,0.199354920578408,
-0.143787277896795));
#37567=CARTESIAN_POINT('Ctrl Pts',(-0.230778801644068,0.00996300771099484,
-0.132667632155194));
#37568=CARTESIAN_POINT('Ctrl Pts',(-0.133432807776802,-0.188557168465927,
-0.121547986413595));
#37569=CARTESIAN_POINT('Ctrl Pts',(0.0861633714242763,-0.214321848634489,
-0.110428340671994));
#37570=CARTESIAN_POINT('Ctrl Pts',(0.226817615214866,-0.0437267120554264,
-0.0993086949303942));
#37571=CARTESIAN_POINT('Ctrl Pts',(0.159661783589004,0.166932042100053,
-0.0881890491887944));
#37572=CARTESIAN_POINT('Ctrl Pts',(-0.0537735371994615,0.224645800138481,
-0.0770694034471939));
#37573=CARTESIAN_POINT('Ctrl Pts',(-0.217945268389443,0.0765454247822962,
-0.0659497577055941));
#37574=CARTESIAN_POINT('Ctrl Pts',(-0.182430110498917,-0.141695345732293,
-0.0548301119639939));
#37575=CARTESIAN_POINT('Ctrl Pts',(0.0202140745200903,-0.230096774851241,
-0.0437104662223939));
#37576=CARTESIAN_POINT('Ctrl Pts',(0.204362022504145,-0.107720528503693,
-0.0325908204807937));
#37577=CARTESIAN_POINT('Ctrl Pts',(0.201229224832426,0.113416905860893,
-0.0214711747391938));
#37578=CARTESIAN_POINT('Ctrl Pts',(0.0138176799773481,0.230512184838331,
-0.0103515289975936));
#37579=CARTESIAN_POINT('Ctrl Pts',(-0.186419316548585,0.136664056575899,
0.000768116744006414));
#37580=CARTESIAN_POINT('Ctrl Pts',(-0.215533805916768,-0.082896432813855,
0.0118877624856065));
#37581=CARTESIAN_POINT('Ctrl Pts',(-0.103772619141881,-0.17787249415385,
0.0193008596466731));
#37582=CARTESIAN_POINT('Ctrl Pts',(-0.0401504189376312,-0.191230499291124,
0.0230074082272065));
#37583=CARTESIAN_POINT('',(-0.149577339797456,0.126231096176531,2.3740120150659E-16));
#37584=CARTESIAN_POINT('Ctrl Pts',(-0.149579224365402,0.126232117338717,
3.12250225675825E-17));
#37585=CARTESIAN_POINT('Ctrl Pts',(-0.15213626770352,0.122550735753821,
1.75395509689456E-17));
#37586=CARTESIAN_POINT('Ctrl Pts',(-0.154553778983314,0.118780419069818,
-2.56435089757285E-17));
#37587=CARTESIAN_POINT('Ctrl Pts',(-0.156823814682293,0.114924149748616,
-7.28583859910259E-17));
#37588=CARTESIAN_POINT('Ctrl Pts',(-0.161285099186592,0.107345451944513,
-1.65588310206067E-16));
#37589=CARTESIAN_POINT('Ctrl Pts',(-0.165177482683705,0.0994348489301857,
-4.45014344919782E-16));
#37590=CARTESIAN_POINT('Ctrl Pts',(-0.168497913306379,0.0912613466614302,
-6.1409211049579E-16));
#37591=CARTESIAN_POINT('Ctrl Pts',(-0.170168203952632,0.0871497942942736,
-6.9914403370195E-16));
#37592=CARTESIAN_POINT('Ctrl Pts',(-0.171694353287266,0.0829692560081717,
-3.2424756013121E-16));
#37593=CARTESIAN_POINT('Ctrl Pts',(-0.173072321343778,0.0787365486429996,
-3.08780778723872E-16));
#37594=CARTESIAN_POINT('Ctrl Pts',(-0.17688112264392,0.0670370457122868,
-2.66029499508873E-16));
#37595=CARTESIAN_POINT('Ctrl Pts',(-0.179552067097139,0.0549719351495626,
-1.72155562539013E-16));
#37596=CARTESIAN_POINT('Ctrl Pts',(-0.181069928572971,0.0427320571800164,
1.45716771982052E-16));
#37597=CARTESIAN_POINT('Ctrl Pts',(-0.181571983366965,0.0386835392418783,
2.50857677107766E-16));
#37598=CARTESIAN_POINT('Ctrl Pts',(-0.181947631644738,0.0346138283481453,
-4.72643688963084E-17));
#37599=CARTESIAN_POINT('Ctrl Pts',(-0.18219485039693,0.0305368171567139,
-6.93889390390723E-17));
#37600=CARTESIAN_POINT('Ctrl Pts',(-0.182940753710731,0.0182357431842819,
-1.36142735179339E-16));
#37601=CARTESIAN_POINT('Ctrl Pts',(-0.182518848032763,0.00592920171664246,
-2.46842689824824E-16));
#37602=CARTESIAN_POINT('Ctrl Pts',(-0.180911458839137,-0.00619024109343332,
-3.34801630863524E-16));
#37603=CARTESIAN_POINT('Ctrl Pts',(-0.179850463364892,-0.0141899676206825,
-3.92861022286291E-16));
#37604=CARTESIAN_POINT('Ctrl Pts',(-0.178271908795443,-0.0221081540245901,
-2.21255589905061E-16));
#37605=CARTESIAN_POINT('Ctrl Pts',(-0.176159106007433,-0.0298838204643374,
-3.40005801291454E-16));
#37606=CARTESIAN_POINT('Ctrl Pts',(-0.174809572472798,-0.0348504565716565,
-4.15856417080292E-16));
#37607=CARTESIAN_POINT('Ctrl Pts',(-0.173239451433683,-0.0397640700380695,
-3.63363244663589E-16));
#37608=CARTESIAN_POINT('Ctrl Pts',(-0.171455092377085,-0.0445771192033741,
-3.71230823859037E-16));
#37609=CARTESIAN_POINT('Ctrl Pts',(-0.169157099318569,-0.0507756214225697,
-3.81363113272206E-16));
#37610=CARTESIAN_POINT('Ctrl Pts',(-0.1665024797364,-0.0568161660521192,
-2.09853073085683E-16));
#37611=CARTESIAN_POINT('Ctrl Pts',(-0.16348481359929,-0.0626658509200692,
-2.98372437868011E-16));
#37612=CARTESIAN_POINT('Ctrl Pts',(-0.158069190177679,-0.0731639275596034,
-4.56902188558693E-16));
#37613=CARTESIAN_POINT('Ctrl Pts',(-0.15148551162908,-0.0830500140735381,
-1.69238594609806E-16));
#37614=CARTESIAN_POINT('Ctrl Pts',(-0.143886948956133,-0.0921970824958435,
-6.24500451351651E-17));
#37615=CARTESIAN_POINT('Ctrl Pts',(-0.141498396059732,-0.0950723969091165,
-2.88818414986653E-17));
#37616=CARTESIAN_POINT('Ctrl Pts',(-0.139008411786517,-0.0978749248249702,
-3.46133223658663E-16));
#37617=CARTESIAN_POINT('Ctrl Pts',(-0.136433692072541,-0.100588045776136,
-3.48679418671338E-16));
#37618=CARTESIAN_POINT('Ctrl Pts',(-0.129595227249087,-0.107794104783498,
-3.55442121785516E-16));
#37619=CARTESIAN_POINT('Ctrl Pts',(-0.122142516767232,-0.114393608368861,
-2.3081146500224E-16));
#37620=CARTESIAN_POINT('Ctrl Pts',(-0.114172290333582,-0.1203153298124,
-2.60208521396521E-16));
#37621=CARTESIAN_POINT('Ctrl Pts',(-0.109745931829009,-0.123604027102437,
-2.76534520621699E-16));
#37622=CARTESIAN_POINT('Ctrl Pts',(-0.105159682538236,-0.126683244398258,
1.53094208316784E-16));
#37623=CARTESIAN_POINT('Ctrl Pts',(-0.100428978517873,-0.129537077171602,
2.34187669256869E-16));
#37624=CARTESIAN_POINT('Ctrl Pts',(-0.0974655015542694,-0.131324816934094,
2.84987423872767E-16));
#37625=CARTESIAN_POINT('Ctrl Pts',(-0.0944453272369587,-0.133024055864704,
-1.57159659481818E-16));
#37626=CARTESIAN_POINT('Ctrl Pts',(-0.091372239374377,-0.134630282149142,
-1.76941794549634E-16));
#37627=CARTESIAN_POINT('Ctrl Pts',(-0.0882085618680696,-0.136283857378145,
-1.97307074860303E-16));
#37628=CARTESIAN_POINT('Ctrl Pts',(-0.084995963230153,-0.137835002018624,
-1.14607397771812E-16));
#37629=CARTESIAN_POINT('Ctrl Pts',(-0.0817435159838432,-0.139278121880328,
-1.25333771139324E-16));
#37630=CARTESIAN_POINT('Ctrl Pts',(-0.0719268932182113,-0.143633784621363,
-1.57708396465424E-16));
#37631=CARTESIAN_POINT('Ctrl Pts',(-0.0617342162816699,-0.147015917264351,
-2.37152691385054E-16));
#37632=CARTESIAN_POINT('Ctrl Pts',(-0.0512859179194202,-0.149305219054896,
-1.346579098227E-16));
#37633=CARTESIAN_POINT('Ctrl Pts',(-0.0449298836761154,-0.150697874592619,
-7.23070543260647E-17));
#37634=CARTESIAN_POINT('Ctrl Pts',(-0.0384791302638158,-0.151685198677283,
-1.58142429239726E-16));
#37635=CARTESIAN_POINT('Ctrl Pts',(-0.0319621170202069,-0.15223082991164,
-1.59594559789866E-16));
#37636=CARTESIAN_POINT('Ctrl Pts',(-0.195209575558751,0.00014773333329694,
-0.0621869692124235));
#37637=CARTESIAN_POINT('Ctrl Pts',(-0.194905259338105,-0.0429573617160955,
-0.059734683462947));
#37638=CARTESIAN_POINT('Ctrl Pts',(-0.180836665151344,-0.0862425843964161,
-0.0572823977134706));
#37639=CARTESIAN_POINT('Ctrl Pts',(-0.154575272644172,-0.120055455499684,
-0.0548301119639941));
#37640=CARTESIAN_POINT('Ctrl Pts',(-0.114882048825917,-0.171162488771942,
-0.0511235633834607));
#37641=CARTESIAN_POINT('Ctrl Pts',(-0.0473339871529112,-0.200629631811592,
-0.0474170148029272));
#37642=CARTESIAN_POINT('Ctrl Pts',(0.0171313683475999,-0.194967162273492,
-0.0437104662223938));
#37643=CARTESIAN_POINT('Ctrl Pts',(0.0815967238481101,-0.189304692735391,
-0.0400039176418604));
#37644=CARTESIAN_POINT('Ctrl Pts',(0.142979373176127,-0.148512610619542,
-0.0362973690613271));
#37645=CARTESIAN_POINT('Ctrl Pts',(0.173148564894849,-0.0912603305008528,
-0.0325908204807937));
#37646=CARTESIAN_POINT('Ctrl Pts',(0.203317756613572,-0.0340080503821637,
-0.0288842719002604));
#37647=CARTESIAN_POINT('Ctrl Pts',(0.202273490722998,0.0397044277393669,
-0.025177723319727));
#37648=CARTESIAN_POINT('Ctrl Pts',(0.170516100301865,0.096076546629704,
-0.0214711747391936));
#37649=CARTESIAN_POINT('Ctrl Pts',(0.138758709880731,0.15244866552004,-0.0177646261586603));
#37650=CARTESIAN_POINT('Ctrl Pts',(0.0762881949290407,0.191480425179185,
-0.014058077578127));
#37651=CARTESIAN_POINT('Ctrl Pts',(0.0116801046988732,0.195354950298353,
-0.0103515289975937));
#37652=CARTESIAN_POINT('Ctrl Pts',(-0.0484650235757366,0.198961833112337,
-0.00690101933172905));
#37653=CARTESIAN_POINT('Ctrl Pts',(-0.110462610495604,0.172100865870811,
-0.00345050966586447));
#37654=CARTESIAN_POINT('Ctrl Pts',(-0.149579224365404,0.126232117338714,
1.70002900645727E-16));
#37655=CARTESIAN_POINT('',(-0.141301845044904,0.0650353064643039,-1.));
#37656=CARTESIAN_POINT('Ctrl Pts',(-0.141514759450945,0.0651925368729976,
-1.));
#37657=CARTESIAN_POINT('Ctrl Pts',(-0.140439543113019,0.0686377703387253,
-1.));
#37658=CARTESIAN_POINT('Ctrl Pts',(-0.139238142539461,0.0720367067892421,
-1.));
#37659=CARTESIAN_POINT('Ctrl Pts',(-0.137910622472938,0.0753822101626856,
-1.));
#37660=CARTESIAN_POINT('Ctrl Pts',(-0.134668353041792,0.0835531023345245,
-1.));
#37661=CARTESIAN_POINT('Ctrl Pts',(-0.130675558679426,0.0914056054140095,
-1.));
#37662=CARTESIAN_POINT('Ctrl Pts',(-0.126026137664389,0.0988943536247196,
-1.));
#37663=CARTESIAN_POINT('Ctrl Pts',(-0.123780053918212,0.102512084860693,
-1.));
#37664=CARTESIAN_POINT('Ctrl Pts',(-0.121379830696976,0.106044927785419,
-1.));
#37665=CARTESIAN_POINT('Ctrl Pts',(-0.118844566172191,0.109475158254566,
-1.));
#37666=CARTESIAN_POINT('Ctrl Pts',(-0.1142132117073,0.115741412936701,-1.));
#37667=CARTESIAN_POINT('Ctrl Pts',(-0.109125681139024,0.121676187684083,
-1.));
#37668=CARTESIAN_POINT('Ctrl Pts',(-0.103641429786816,0.127248528569788,
-1.));
#37669=CARTESIAN_POINT('Ctrl Pts',(-0.100783730165235,0.130152129338194,
-1.));
#37670=CARTESIAN_POINT('Ctrl Pts',(-0.0978169100852653,0.132958315023231,
-1.));
#37671=CARTESIAN_POINT('Ctrl Pts',(-0.0947519441241897,0.135658875758607,
-1.));
#37672=CARTESIAN_POINT('Ctrl Pts',(-0.0860010566744776,0.14336933758641,
-1.));
#37673=CARTESIAN_POINT('Ctrl Pts',(-0.0765074634433449,0.150174174108871,
-1.));
#37674=CARTESIAN_POINT('Ctrl Pts',(-0.0664560352410665,0.155977668638949,
-1.));
#37675=CARTESIAN_POINT('Ctrl Pts',(-0.0587959349774297,0.16040045802621,
-1.));
#37676=CARTESIAN_POINT('Ctrl Pts',(-0.0508104927247559,0.164241610466299,
-1.));
#37677=CARTESIAN_POINT('Ctrl Pts',(-0.0425661446334144,0.167446298872687,
-1.));
#37678=CARTESIAN_POINT('Ctrl Pts',(-0.0392699210733563,0.168727585071517,
-1.));
#37679=CARTESIAN_POINT('Ctrl Pts',(-0.0359322471339816,0.169906628237342,
-1.));
#37680=CARTESIAN_POINT('Ctrl Pts',(-0.0325709935602962,0.170975746975499,
-1.));
#37681=CARTESIAN_POINT('Ctrl Pts',(-0.0260409344851832,0.173052772217845,
-1.));
#37682=CARTESIAN_POINT('Ctrl Pts',(-0.0194097376667411,0.174720258844212,
-1.));
#37683=CARTESIAN_POINT('Ctrl Pts',(-0.0127103276648721,0.175957707572939,
-1.));
#37684=CARTESIAN_POINT('Ctrl Pts',(-0.00513764342403194,0.17735645887854,
-1.));
#37685=CARTESIAN_POINT('Ctrl Pts',(0.00252225608355841,0.178206122099873,
-1.));
#37686=CARTESIAN_POINT('Ctrl Pts',(0.0102240731002703,0.178534251350247,
-1.));
#37687=CARTESIAN_POINT('Ctrl Pts',(0.0149026548551076,0.178733578277996,
-1.));
#37688=CARTESIAN_POINT('Ctrl Pts',(0.0195967888085301,0.178740260799471,
-1.));
#37689=CARTESIAN_POINT('Ctrl Pts',(0.0242967627079693,0.178558747054534,
-1.));
#37690=CARTESIAN_POINT('Ctrl Pts',(0.0278750965504952,0.178420551228283,
-1.));
#37691=CARTESIAN_POINT('Ctrl Pts',(0.0314562829551843,0.178172985748135,
-1.));
#37692=CARTESIAN_POINT('Ctrl Pts',(0.0350223326126129,0.177819803126781,
-1.));
#37693=CARTESIAN_POINT('Ctrl Pts',(0.0464531859559181,0.176687688003343,
-1.));
#37694=CARTESIAN_POINT('Ctrl Pts',(0.057763458181646,0.174472683704982,
-1.));
#37695=CARTESIAN_POINT('Ctrl Pts',(0.0688115888091587,0.171259810959209,
-1.));
#37696=CARTESIAN_POINT('Ctrl Pts',(0.0755835048896587,0.169290490958818,
-1.));
#37697=CARTESIAN_POINT('Ctrl Pts',(0.0822572209906249,0.16694544858736,
-1.));
#37698=CARTESIAN_POINT('Ctrl Pts',(0.0888005398454858,0.164236932162052,
-1.));
#37699=CARTESIAN_POINT('Ctrl Pts',(0.0937380717004385,0.162193109076817,
-1.));
#37700=CARTESIAN_POINT('Ctrl Pts',(0.0986065782001952,0.159939028720903,
-1.));
#37701=CARTESIAN_POINT('Ctrl Pts',(0.103361681203228,0.157494885851826,
-1.));
#37702=CARTESIAN_POINT('Ctrl Pts',(0.114767902239668,0.151632040443103,
-1.));
#37703=CARTESIAN_POINT('Ctrl Pts',(0.125550646082581,0.144670357618447,
-1.));
#37704=CARTESIAN_POINT('Ctrl Pts',(0.135527553857112,0.13669485551301,-1.));
#37705=CARTESIAN_POINT('Ctrl Pts',(0.142856934691975,0.130835776367343,
-1.));
#37706=CARTESIAN_POINT('Ctrl Pts',(0.149751664752612,0.124428399142311,
-1.));
#37707=CARTESIAN_POINT('Ctrl Pts',(0.156132246633335,0.117489921104865,
-1.));
#37708=CARTESIAN_POINT('Ctrl Pts',(-0.141514759450946,0.0651925368729961,
-1.));
#37709=CARTESIAN_POINT('Ctrl Pts',(-0.150731766956786,0.0449100614655458,
-0.99839812581321));
#37710=CARTESIAN_POINT('Ctrl Pts',(-0.15533019555488,0.0224563452055557,
-0.996796251626419));
#37711=CARTESIAN_POINT('Ctrl Pts',(-0.155319281545194,2.55672115836644E-6,
-0.995194377439629));
#37712=CARTESIAN_POINT('Origin',(-2.59090492670967E-17,0.,-1.));
#37713=CARTESIAN_POINT('Ctrl Pts',(0.188715001522267,-0.051914696198531,
-1.));
#37714=CARTESIAN_POINT('Ctrl Pts',(0.187126268659119,-0.0561059924632036,
-1.));
#37715=CARTESIAN_POINT('Ctrl Pts',(0.185385258844343,-0.0602325559568805,
-1.));
#37716=CARTESIAN_POINT('Ctrl Pts',(0.183489936934311,-0.0642861493789803,
-1.));
#37717=CARTESIAN_POINT('Ctrl Pts',(0.179765074014344,-0.0722526482363455,
-1.));
#37718=CARTESIAN_POINT('Ctrl Pts',(0.17544466132878,-0.0799378474501277,
-1.));
#37719=CARTESIAN_POINT('Ctrl Pts',(0.170583870709489,-0.0873001880106591,
-1.));
#37720=CARTESIAN_POINT('Ctrl Pts',(0.16813872456559,-0.0910037004722348,
-1.));
#37721=CARTESIAN_POINT('Ctrl Pts',(0.165555142410874,-0.094627392494239,
-1.));
#37722=CARTESIAN_POINT('Ctrl Pts',(0.162844704799912,-0.098158418110447,
-1.));
#37723=CARTESIAN_POINT('Ctrl Pts',(0.155352865708622,-0.107918419830045,
-1.));
#37724=CARTESIAN_POINT('Ctrl Pts',(0.146915777629002,-0.116947057395722,
-1.));
#37725=CARTESIAN_POINT('Ctrl Pts',(0.137682182322815,-0.125123801279632,
-1.));
#37726=CARTESIAN_POINT('Ctrl Pts',(0.134628037165296,-0.127828377548053,
-1.));
#37727=CARTESIAN_POINT('Ctrl Pts',(0.131484897843174,-0.130440716087263,
-1.));
#37728=CARTESIAN_POINT('Ctrl Pts',(0.12826307503258,-0.132951288440458,
-1.));
#37729=CARTESIAN_POINT('Ctrl Pts',(0.118542257931425,-0.140526135382502,
-1.));
#37730=CARTESIAN_POINT('Ctrl Pts',(0.10815619820295,-0.147141159084441,
-1.));
#37731=CARTESIAN_POINT('Ctrl Pts',(0.0972536752672356,-0.15267283480508,
-1.));
#37732=CARTESIAN_POINT('Ctrl Pts',(0.090057189388818,-0.156324157204702,
-1.));
#37733=CARTESIAN_POINT('Ctrl Pts',(0.0826351063399878,-0.159502589968769,
-1.));
#37734=CARTESIAN_POINT('Ctrl Pts',(0.0750282645074606,-0.162159870196947,
-1.));
#37735=CARTESIAN_POINT('Ctrl Pts',(0.0701695094492505,-0.163857167713314,
-1.));
#37736=CARTESIAN_POINT('Ctrl Pts',(0.0652296690239961,-0.165342583374345,
-1.));
#37737=CARTESIAN_POINT('Ctrl Pts',(0.0602515354147416,-0.166594454550118,
-1.));
#37738=CARTESIAN_POINT('Ctrl Pts',(0.0538403798350176,-0.168206693494195,
-1.));
#37739=CARTESIAN_POINT('Ctrl Pts',(0.0473576918062638,-0.169435505552497,
-1.));
#37740=CARTESIAN_POINT('Ctrl Pts',(0.0408269682982621,-0.170256981483823,
-1.));
#37741=CARTESIAN_POINT('Ctrl Pts',(0.0291066787191395,-0.171731234035722,
-1.));
#37742=CARTESIAN_POINT('Ctrl Pts',(0.017230129317074,-0.171896111652057,
-1.));
#37743=CARTESIAN_POINT('Ctrl Pts',(0.00538872457353722,-0.170806039426225,
-1.));
#37744=CARTESIAN_POINT('Ctrl Pts',(0.00166646623728207,-0.170463383253449,
-1.));
#37745=CARTESIAN_POINT('Ctrl Pts',(-0.0020531649922566,-0.169995910229923,
-1.));
#37746=CARTESIAN_POINT('Ctrl Pts',(-0.00574701830086723,-0.169407983257621,
-1.));
#37747=CARTESIAN_POINT('Ctrl Pts',(-0.0155579084828646,-0.167846446705308,
-1.));
#37748=CARTESIAN_POINT('Ctrl Pts',(-0.0252161982402266,-0.165435252063536,
-1.));
#37749=CARTESIAN_POINT('Ctrl Pts',(-0.0346084283051884,-0.162213857880575,
-1.));
#37750=CARTESIAN_POINT('Ctrl Pts',(-0.0398245124126221,-0.160424819187389,
-1.));
#37751=CARTESIAN_POINT('Ctrl Pts',(-0.0449583344912096,-0.158385421116544,
-1.));
#37752=CARTESIAN_POINT('Ctrl Pts',(-0.0499880468050878,-0.156099392746595,
-1.));
#37753=CARTESIAN_POINT('Ctrl Pts',(-0.0531388312209868,-0.154667346117912,
-1.));
#37754=CARTESIAN_POINT('Ctrl Pts',(-0.0562487211166722,-0.153138476967067,
-1.));
#37755=CARTESIAN_POINT('Ctrl Pts',(-0.0593118554215172,-0.151513352468256,
-1.));
#37756=CARTESIAN_POINT('Ctrl Pts',(-0.0624652902574377,-0.149840319653745,
-1.));
#37757=CARTESIAN_POINT('Ctrl Pts',(-0.0655619449577883,-0.14806899457065,
-1.));
#37758=CARTESIAN_POINT('Ctrl Pts',(-0.0685920735998228,-0.146203692832195,
-1.));
#37759=CARTESIAN_POINT('Ctrl Pts',(-0.0777376759071703,-0.140573797240811,
-1.));
#37760=CARTESIAN_POINT('Ctrl Pts',(-0.086293321868111,-0.13408301355852,
-1.));
#37761=CARTESIAN_POINT('Ctrl Pts',(-0.0940925019796224,-0.126763144612894,
-1.));
#37762=CARTESIAN_POINT('Ctrl Pts',(-0.0988370020441118,-0.122310225435747,
-1.));
#37763=CARTESIAN_POINT('Ctrl Pts',(-0.103300876049684,-0.117549871947081,
-1.));
#37764=CARTESIAN_POINT('Ctrl Pts',(-0.107438039834494,-0.112484977203721,
-1.));
#37765=CARTESIAN_POINT('Origin',(0.,0.,-1.));
#37766=CARTESIAN_POINT('Origin',(0.,0.,-1.18400562256037));
#37767=CARTESIAN_POINT('Ctrl Pts',(-0.134962346407334,-0.141302247159154,
-1.02300740822721));
#37768=CARTESIAN_POINT('Ctrl Pts',(-0.0879512268871996,-0.186204087895818,
-1.01930085964667));
#37769=CARTESIAN_POINT('Ctrl Pts',(0.0535947059270241,-0.224620144876903,
-1.01188776248561));
#37770=CARTESIAN_POINT('Ctrl Pts',(0.218160338720414,-0.0763889482965145,
-1.00076811674401));
#37771=CARTESIAN_POINT('Ctrl Pts',(0.182250900350768,0.141814812868076,
-0.989648471002405));
#37772=CARTESIAN_POINT('Ctrl Pts',(-0.020335578424721,0.230093582492485,
-0.978528825260807));
#37773=CARTESIAN_POINT('Ctrl Pts',(-0.204446822720336,0.107559487262165,
-0.967409179519207));
#37774=CARTESIAN_POINT('Ctrl Pts',(-0.201163147192314,-0.113518873259326,
-0.956289533777606));
#37775=CARTESIAN_POINT('Ctrl Pts',(-0.0136177717725777,-0.23059244536116,
-0.945169888036007));
#37776=CARTESIAN_POINT('Ctrl Pts',(0.186426678942524,-0.136398090256529,
-0.934050242294405));
#37777=CARTESIAN_POINT('Ctrl Pts',(0.215656133902945,0.0827633194859286,
-0.922930596552807));
#37778=CARTESIAN_POINT('Ctrl Pts',(0.0473087718922573,0.226097493403868,
-0.911810950811205));
#37779=CARTESIAN_POINT('Ctrl Pts',(-0.164385906299704,0.16228226783603,
-0.900691305069606));
#37780=CARTESIAN_POINT('Ctrl Pts',(-0.225469354113307,-0.0502151067302932,
-0.889571659328005));
#37781=CARTESIAN_POINT('Ctrl Pts',(-0.0799798472802848,-0.216705673394779,
-0.878452013586406));
#37782=CARTESIAN_POINT('Ctrl Pts',(0.138787254209544,-0.184651617385904,
-0.867332367844805));
#37783=CARTESIAN_POINT('Ctrl Pts',(0.230397943777862,0.0165792908334795,
-0.856212722103206));
#37784=CARTESIAN_POINT('Ctrl Pts',(0.110919360557233,0.202620340500548,
-0.845093076361604));
#37785=CARTESIAN_POINT('Ctrl Pts',(-0.110183034939153,0.203021682345978,
-0.833973430620007));
#37786=CARTESIAN_POINT('Ctrl Pts',(-0.230336268383591,0.0174156105429483,
-0.822853784878404));
#37787=CARTESIAN_POINT('Ctrl Pts',(-0.139456624242068,-0.18414655373536,
-0.811734139136807));
#37788=CARTESIAN_POINT('Ctrl Pts',(0.079192466865668,-0.21699459881069,
-0.800614493395203));
#37789=CARTESIAN_POINT('Ctrl Pts',(0.225285824667576,-0.0510333160814544,
-0.789494847653607));
#37790=CARTESIAN_POINT('Ctrl Pts',(0.164973479123837,0.161684426641202,
-0.778375201912004));
#37791=CARTESIAN_POINT('Ctrl Pts',(-0.0464867152313373,0.226267734821794,
-0.767255556170406));
#37792=CARTESIAN_POINT('Ctrl Pts',(-0.215356021036036,0.083545715935049,
-0.756135910428805));
#37793=CARTESIAN_POINT('Ctrl Pts',(-0.18691725583042,-0.135720455315325,
-0.745016264687205));
#37794=CARTESIAN_POINT('Ctrl Pts',(0.0127741315575716,-0.230640248134116,
-0.733896618945605));
#37795=CARTESIAN_POINT('Ctrl Pts',(0.200761925645074,-0.114248639819529,
-0.722776973204004));
#37796=CARTESIAN_POINT('Ctrl Pts',(0.204812683015893,0.106816980743676,
-0.711657327462405));
#37797=CARTESIAN_POINT('Ctrl Pts',(0.0212151206534201,0.230017436624418,
-0.700537681720805));
#37798=CARTESIAN_POINT('Ctrl Pts',(-0.181819625388585,0.142477108050848,
-0.689418035979204));
#37799=CARTESIAN_POINT('Ctrl Pts',(-0.218272172080734,-0.0756000092032434,
-0.678298390237605));
#37800=CARTESIAN_POINT('Ctrl Pts',(-0.0547448848744599,-0.224412789465829,
-0.667178744496004));
#37801=CARTESIAN_POINT('Ctrl Pts',(0.15893938239428,-0.167619733980953,
-0.656059098754404));
#37802=CARTESIAN_POINT('Ctrl Pts',(0.227004210468479,0.0427456538784019,
-0.644939453012805));
#37803=CARTESIAN_POINT('Ctrl Pts',(0.0870889562897442,0.213947694982147,
-0.633819807271204));
#37804=CARTESIAN_POINT('Ctrl Pts',(-0.132616748713462,0.189131965718346,
-0.622700161529604));
#37805=CARTESIAN_POINT('Ctrl Pts',(-0.230819675206534,-0.00896549125201681,
-0.611580515788004));
#37806=CARTESIAN_POINT('Ctrl Pts',(-0.117546810409861,-0.198848811558663,
-0.600460870046404));
#37807=CARTESIAN_POINT('Ctrl Pts',(0.103421833452207,-0.206547880311589,
-0.589341224304804));
#37808=CARTESIAN_POINT('Ctrl Pts',(0.229635929001371,-0.0250088505834818,
-0.578221578563204));
#37809=CARTESIAN_POINT('Ctrl Pts',(0.145458775404855,0.179443158558768,
-0.567101932821604));
#37810=CARTESIAN_POINT('Ctrl Pts',(-0.0719869550633662,0.219490274947508,
-0.555982287080004));
#37811=CARTESIAN_POINT('Ctrl Pts',(-0.223478610035487,0.0584415379027191,
-0.544862641338404));
#37812=CARTESIAN_POINT('Ctrl Pts',(-0.17022031961721,-0.156151033570842,
-0.533742995596803));
#37813=CARTESIAN_POINT('Ctrl Pts',(0.0389929462701933,-0.227678836603225,
-0.522623349855203));
#37814=CARTESIAN_POINT('Ctrl Pts',(0.212481076681926,-0.0906084684117187,
-0.511503704113604));
#37815=CARTESIAN_POINT('Ctrl Pts',(0.191295144818936,0.129476909387466,
-0.500384058372003));
#37816=CARTESIAN_POINT('Ctrl Pts',(-0.00515440824209666,0.230936213209409,
-0.489264412630403));
#37817=CARTESIAN_POINT('Ctrl Pts',(-0.196881519160137,0.120812954226874,
-0.478144766888803));
#37818=CARTESIAN_POINT('Ctrl Pts',(-0.208226801633768,-0.0999985078748647,
-0.467025121147203));
#37819=CARTESIAN_POINT('Ctrl Pts',(-0.0287957666040805,-0.229191854832389,
-0.455905475405603));
#37820=CARTESIAN_POINT('Ctrl Pts',(0.177017800689991,-0.148400811098552,
-0.444785829664003));
#37821=CARTESIAN_POINT('Ctrl Pts',(0.220648575551937,0.0683542873763441,
-0.433666183922403));
#37822=CARTESIAN_POINT('Ctrl Pts',(0.0621222679640238,0.222483541680797,
-0.422546538180802));
#37823=CARTESIAN_POINT('Ctrl Pts',(-0.153320139876834,0.172774527069206,
-0.411426892439203));
#37824=CARTESIAN_POINT('Ctrl Pts',(-0.228291429421142,-0.0352296146539616,
-0.400307246697602));
#37825=CARTESIAN_POINT('Ctrl Pts',(-0.0941032933737792,-0.210956565842401,
-0.389187600956003));
#37826=CARTESIAN_POINT('Ctrl Pts',(0.126301792816278,-0.193406203693944,
-0.378067955214402));
#37827=CARTESIAN_POINT('Ctrl Pts',(0.230989830391116,0.00134192086369089,
-0.366948309472803));
#37828=CARTESIAN_POINT('Ctrl Pts',(0.124046181378033,0.194860584473312,
-0.355828663731202));
#37829=CARTESIAN_POINT('Ctrl Pts',(-0.0965479367307507,0.209848989536302,
-0.344709017989603));
#37830=CARTESIAN_POINT('Ctrl Pts',(-0.228685335108273,0.0325748369358222,
-0.333589372248002));
#37831=CARTESIAN_POINT('Ctrl Pts',(-0.151302413548674,-0.174544212593695,
-0.322469726506402));
#37832=CARTESIAN_POINT('Ctrl Pts',(0.0647029959036807,-0.221746758308778,
-0.311350080764802));
#37833=CARTESIAN_POINT('Ctrl Pts',(0.22142785550674,-0.065786072196304,
-0.300230435023202));
#37834=CARTESIAN_POINT('Ctrl Pts',(0.175281660439362,0.15044747259438,-0.289110789281602));
#37835=CARTESIAN_POINT('Ctrl Pts',(-0.031456684426298,0.228841822058552,
-0.277991143540001));
#37836=CARTESIAN_POINT('Ctrl Pts',(-0.209374577754782,0.0975724788943068,
-0.266871497798402));
#37837=CARTESIAN_POINT('Ctrl Pts',(-0.195464567310726,-0.123092263934074,
-0.255751852056802));
#37838=CARTESIAN_POINT('Ctrl Pts',(-0.0024709318560192,-0.230980512442675,
-0.244632206315202));
#37839=CARTESIAN_POINT('Ctrl Pts',(0.192786557592405,-0.127245610368647,
-0.233512560573602));
#37840=CARTESIAN_POINT('Ctrl Pts',(0.211414003045909,0.0930710590752383,
-0.222392914832001));
#37841=CARTESIAN_POINT('Ctrl Pts',(0.0363450300153787,0.228116509904006,
-0.211273269090402));
#37842=CARTESIAN_POINT('Ctrl Pts',(-0.172023064569064,0.154162788245832,
-0.200153623348801));
#37843=CARTESIAN_POINT('Ctrl Pts',(-0.222784530965761,-0.0610340679732166,
-0.189033977607201));
#37844=CARTESIAN_POINT('Ctrl Pts',(-0.0694319391096267,-0.220311853431586,
-0.177914331865601));
#37845=CARTESIAN_POINT('Ctrl Pts',(0.147533789176124,-0.17774100942929,
-0.166794686124001));
#37846=CARTESIAN_POINT('Ctrl Pts',(0.229329912608031,0.0276751317512237,
-0.155675040382401));
#37847=CARTESIAN_POINT('Ctrl Pts',(0.10101498825337,0.207735642104657,-0.144555394640801));
#37848=CARTESIAN_POINT('Ctrl Pts',(-0.119849022951734,0.197469486973865,
-0.133435748899201));
#37849=CARTESIAN_POINT('Ctrl Pts',(-0.230908593740765,0.00628346883829749,
-0.122316103157601));
#37850=CARTESIAN_POINT('Ctrl Pts',(-0.130409737561855,-0.19066068491043,
-0.111196457416001));
#37851=CARTESIAN_POINT('Ctrl Pts',(0.0895676188451145,-0.212920118346556,
-0.100076811674401));
#37852=CARTESIAN_POINT('Ctrl Pts',(0.227487825795308,-0.0401077892944868,
-0.0889571659328005));
#37853=CARTESIAN_POINT('Ctrl Pts',(0.156976791925724,0.169459748502108,
-0.0778375201912006));
#37854=CARTESIAN_POINT('Ctrl Pts',(-0.0573401927066776,0.223752650654119,
-0.0667178744496004));
#37855=CARTESIAN_POINT('Ctrl Pts',(-0.219151667511382,0.0730759416464898,
-0.0555982287080003));
#37856=CARTESIAN_POINT('Ctrl Pts',(-0.180121743363499,-0.144612413097174,
-0.0444785829664003));
#37857=CARTESIAN_POINT('Ctrl Pts',(0.0238283851653625,-0.229693360565524,
-0.0333589372248002));
#37858=CARTESIAN_POINT('Ctrl Pts',(0.206151341171209,-0.104550606625525,
-0.0222392914832002));
#37859=CARTESIAN_POINT('Ctrl Pts',(0.199196267801896,0.116822296166958,
-0.0111196457416001));
#37860=CARTESIAN_POINT('Ctrl Pts',(0.0734855601112398,0.192372693268079,
-0.00370654858053334));
#37861=CARTESIAN_POINT('Ctrl Pts',(0.00853826423430722,0.195213365433479,
0.));
#37862=CARTESIAN_POINT('Ctrl Pts',(-0.125787577549722,-0.131696490507342,
-1.01533827215147));
#37863=CARTESIAN_POINT('Ctrl Pts',(-0.0819722838789168,-0.173545894612556,
-1.01163172357094));
#37864=CARTESIAN_POINT('Ctrl Pts',(0.049951326481116,-0.209350419913845,
-1.00421862640987));
#37865=CARTESIAN_POINT('Ctrl Pts',(0.20332975274633,-0.0711960114326169,
-0.99309898066827));
#37866=CARTESIAN_POINT('Ctrl Pts',(0.169861445593043,0.132174211890948,
-0.981979334926672));
#37867=CARTESIAN_POINT('Ctrl Pts',(-0.0189531615017859,0.214451772082513,
-0.97085968918507));
#37868=CARTESIAN_POINT('Ctrl Pts',(-0.190548484464784,0.100247570565819,
-0.959740043443472));
#37869=CARTESIAN_POINT('Ctrl Pts',(-0.187488033893757,-0.105801836242295,
-0.948620397701869));
#37870=CARTESIAN_POINT('Ctrl Pts',(-0.0126920327668837,-0.21491672214785,
-0.937500751960273));
#37871=CARTESIAN_POINT('Ctrl Pts',(0.173753353872823,-0.127125719228342,
-0.926381106218669));
#37872=CARTESIAN_POINT('Ctrl Pts',(0.200995784302071,0.0771370515201939,
-0.915261460477071));
#37873=CARTESIAN_POINT('Ctrl Pts',(0.0440927115717062,0.210727337975441,
-0.904141814735469));
#37874=CARTESIAN_POINT('Ctrl Pts',(-0.153210917616587,0.151250284940659,
-0.893022168993871));
#37875=CARTESIAN_POINT('Ctrl Pts',(-0.210141899726723,-0.0468014731526719,
-0.881902523252271));
#37876=CARTESIAN_POINT('Ctrl Pts',(-0.074542800343881,-0.201973975877239,
-0.87078287751067));
#37877=CARTESIAN_POINT('Ctrl Pts',(0.129352467310449,-0.172098961376302,
-0.85966323176907));
#37878=CARTESIAN_POINT('Ctrl Pts',(0.214735442823328,0.0154522271355718,
-0.84854358602747));
#37879=CARTESIAN_POINT('Ctrl Pts',(0.103379038963568,0.188846166892656,
-0.83742394028587));
#37880=CARTESIAN_POINT('Ctrl Pts',(-0.102692768916763,0.189220225434536,
-0.826304294544271));
#37881=CARTESIAN_POINT('Ctrl Pts',(-0.214677960135406,0.0162316936542803,
-0.815184648802669));
#37882=CARTESIAN_POINT('Ctrl Pts',(-0.129976333426566,-0.171628232059561,
-0.804065003061071));
#37883=CARTESIAN_POINT('Ctrl Pts',(0.0738089462164079,-0.20224326008226,
-0.792945357319469));
#37884=CARTESIAN_POINT('Ctrl Pts',(0.209970846651535,-0.0475640604590616,
-0.78182571157787));
#37885=CARTESIAN_POINT('Ctrl Pts',(0.153758547115844,0.15069308511672,-0.77070606583627));
#37886=CARTESIAN_POINT('Ctrl Pts',(-0.0433265384964888,0.210886006345764,
-0.759586420094669));
#37887=CARTESIAN_POINT('Ctrl Pts',(-0.200716073171338,0.0778662604931993,
-0.74846677435307));
#37888=CARTESIAN_POINT('Ctrl Pts',(-0.174210581240105,-0.126494150053784,
-0.737347128611469));
#37889=CARTESIAN_POINT('Ctrl Pts',(0.0119057433921528,-0.214961275278188,
-0.726227482869869));
#37890=CARTESIAN_POINT('Ctrl Pts',(0.187114087472171,-0.106481993117365,
-0.715107837128269));
#37891=CARTESIAN_POINT('Ctrl Pts',(0.190889473500056,0.0995555397975229,
-0.703988191386669));
#37892=CARTESIAN_POINT('Ctrl Pts',(0.0197729122637246,0.214380802626665,
-0.69286854564507));
#37893=CARTESIAN_POINT('Ctrl Pts',(-0.169459488794018,0.132791484107098,
-0.681748899903469));
#37894=CARTESIAN_POINT('Ctrl Pts',(-0.203433983651159,-0.0704607045857945,
-0.670629254161869));
#37895=CARTESIAN_POINT('Ctrl Pts',(-0.0510233160204035,-0.209157160567478,
-0.659509608420268));
#37896=CARTESIAN_POINT('Ctrl Pts',(0.148134649558368,-0.156224909008006,
-0.648389962678669));
#37897=CARTESIAN_POINT('Ctrl Pts',(0.2115724162222,0.0398397952856799,-0.637270316937069));
#37898=CARTESIAN_POINT('Ctrl Pts',(0.081168630619074,0.199403485420499,
-0.626150671195468));
#37899=CARTESIAN_POINT('Ctrl Pts',(-0.123601434083249,0.176274734681368,
-0.615031025453869));
#37900=CARTESIAN_POINT('Ctrl Pts',(-0.21512850486027,-0.00835601526021841,
-0.603911379712268));
#37901=CARTESIAN_POINT('Ctrl Pts',(-0.109555953373298,-0.185331027286038,
-0.592791733970669));
#37902=CARTESIAN_POINT('Ctrl Pts',(0.0963911953371101,-0.192506711716541,
-0.581672088229068));
#37903=CARTESIAN_POINT('Ctrl Pts',(0.214025229972533,-0.023308743630646,
-0.570552442487468));
#37904=CARTESIAN_POINT('Ctrl Pts',(0.135570457083661,0.167244574681991,
-0.559432796745868));
#37905=CARTESIAN_POINT('Ctrl Pts',(-0.0670932666306222,0.204569279627381,
-0.548313151004268));
#37906=CARTESIAN_POINT('Ctrl Pts',(-0.20828648685242,0.0544686697938416,
-0.537193505262669));
#37907=CARTESIAN_POINT('Ctrl Pts',(-0.158648706282604,-0.145535853277772,
-0.526073859521068));
#37908=CARTESIAN_POINT('Ctrl Pts',(0.0363421975344947,-0.2122011811296,
-0.514954213779468));
#37909=CARTESIAN_POINT('Ctrl Pts',(0.198036568142563,-0.0844488855625077,
-0.503834568037868));
#37910=CARTESIAN_POINT('Ctrl Pts',(0.178290860409118,0.12067504169881,-0.492714922296268));
#37911=CARTESIAN_POINT('Ctrl Pts',(-0.00480401047947801,0.215237120585057,
-0.481595276554667));
#37912=CARTESIAN_POINT('Ctrl Pts',(-0.18349747184091,0.112600064042736,
-0.470475630813068));
#37913=CARTESIAN_POINT('Ctrl Pts',(-0.194071499612093,-0.0932005881566582,
-0.459355985071467));
#37914=CARTESIAN_POINT('Ctrl Pts',(-0.0268382242991108,-0.213611344059494,
-0.448236339329868));
#37915=CARTESIAN_POINT('Ctrl Pts',(0.164984093154174,-0.138312492568566,
-0.437116693588267));
#37916=CARTESIAN_POINT('Ctrl Pts',(0.205648838711703,0.0637075484613892,
-0.425997047846667));
#37917=CARTESIAN_POINT('Ctrl Pts',(0.0578991830469871,0.20735906345497,
-0.414877402105067));
#37918=CARTESIAN_POINT('Ctrl Pts',(-0.142897404335907,0.161029278171717,
-0.403757756363467));
#37919=CARTESIAN_POINT('Ctrl Pts',(-0.212772129758173,-0.0328346979975991,
-0.392638110621867));
#37920=CARTESIAN_POINT('Ctrl Pts',(-0.0877061315843801,-0.196615693872392,
-0.381518464880267));
#37921=CARTESIAN_POINT('Ctrl Pts',(0.11771577022377,-0.180258409055248,
-0.370398819138667));
#37922=CARTESIAN_POINT('Ctrl Pts',(0.21528709285941,0.00125069679951916,
-0.359279173397067));
#37923=CARTESIAN_POINT('Ctrl Pts',(0.115613495728229,0.181613920721587,
-0.348159527655467));
#37924=CARTESIAN_POINT('Ctrl Pts',(-0.0899845875688268,0.195583410837868,
-0.337039881913867));
#37925=CARTESIAN_POINT('Ctrl Pts',(-0.213139257653369,0.0303603926303067,
-0.325920236172267));
#37926=CARTESIAN_POINT('Ctrl Pts',(-0.141016843470348,-0.162678660099908,
-0.314800590430666));
#37927=CARTESIAN_POINT('Ctrl Pts',(0.0603044725554018,-0.206672366772434,
-0.303680944689067));
#37928=CARTESIAN_POINT('Ctrl Pts',(0.206375143050337,-0.0613139210925453,
-0.292561298947466));
#37929=CARTESIAN_POINT('Ctrl Pts',(0.163365976085031,0.140220021582975,
-0.281441653205867));
#37930=CARTESIAN_POINT('Ctrl Pts',(-0.029318252364907,0.213285106587666,
-0.270322007464266));
#37931=CARTESIAN_POINT('Ctrl Pts',(-0.19514124966961,0.0909394811393789,
-0.259202361722666));
#37932=CARTESIAN_POINT('Ctrl Pts',(-0.182176844677951,-0.114724425793896,
-0.248082715981066));
#37933=CARTESIAN_POINT('Ctrl Pts',(-0.00230295738576517,-0.215278408347075,
-0.236963070239466));
#37934=CARTESIAN_POINT('Ctrl Pts',(0.179680886626768,-0.118595426859279,
-0.225843424497866));
#37935=CARTESIAN_POINT('Ctrl Pts',(0.197042034398042,0.0867440687918065,
-0.214723778756266));
#37936=CARTESIAN_POINT('Ctrl Pts',(0.0338742871867991,0.212609101306813,
-0.203604133014666));
#37937=CARTESIAN_POINT('Ctrl Pts',(-0.160328900251294,0.143682769290532,
-0.192484487273066));
#37938=CARTESIAN_POINT('Ctrl Pts',(-0.207639591424673,-0.0568849591217459,
-0.181364841531466));
#37939=CARTESIAN_POINT('Ctrl Pts',(-0.0647119412018833,-0.205335007032323,
-0.170245195789866));
#37940=CARTESIAN_POINT('Ctrl Pts',(0.137504410979829,-0.165658138010392,
-0.159125550048266));
#37941=CARTESIAN_POINT('Ctrl Pts',(0.213740016638345,0.0257937704406031,
-0.148005904306665));
#37942=CARTESIAN_POINT('Ctrl Pts',(0.0941479679840126,0.193613729211668,
-0.136886258565066));
#37943=CARTESIAN_POINT('Ctrl Pts',(-0.111701661019585,0.184045469478285,
-0.125766612823465));
#37944=CARTESIAN_POINT('Ctrl Pts',(-0.215211378693734,0.00585631729751509,
-0.114646967081866));
#37945=CARTESIAN_POINT('Ctrl Pts',(-0.121544456016579,-0.177699531219403,
-0.103527321340265));
#37946=CARTESIAN_POINT('Ctrl Pts',(0.0834787931696162,-0.198445763661959,
-0.0924076755986652));
#37947=CARTESIAN_POINT('Ctrl Pts',(0.212023155276811,-0.0373812532941696,
-0.081288029857065));
#37948=CARTESIAN_POINT('Ctrl Pts',(0.146305476405014,0.157939838952792,
-0.0701683841154652));
#37949=CARTESIAN_POINT('Ctrl Pts',(-0.0534421942771988,0.208541898131829,
-0.0590487383738648));
#37950=CARTESIAN_POINT('Ctrl Pts',(-0.20425369079639,0.0681082236754674,
-0.0479290926322649));
#37951=CARTESIAN_POINT('Ctrl Pts',(-0.167877029148153,-0.134781630664691,
-0.0368094468906647));
#37952=CARTESIAN_POINT('Ctrl Pts',(0.0222085265013588,-0.214078757326807,
-0.0256898011490648));
#37953=CARTESIAN_POINT('Ctrl Pts',(0.192137129390805,-0.0974432342713328,
-0.0145701554074646));
#37954=CARTESIAN_POINT('Ctrl Pts',(0.185654863380358,0.108880691761887,
-0.00345050966586461));
#37955=CARTESIAN_POINT('Ctrl Pts',(0.0684899961903367,0.179295156886754,
0.00396258749520215));
#37956=CARTESIAN_POINT('Ctrl Pts',(0.00795783122554286,0.181942719557457,
0.00766913607573549));
#37957=CARTESIAN_POINT('Ctrl Pts',(-0.116612808692109,-0.122090733855531,
-1.00766913607574));
#37958=CARTESIAN_POINT('Ctrl Pts',(-0.0759933408706338,-0.160887701329294,
-1.0039625874952));
#37959=CARTESIAN_POINT('Ctrl Pts',(0.0463079470352078,-0.194080694950787,
-0.996549490334135));
#37960=CARTESIAN_POINT('Ctrl Pts',(0.188499166772245,-0.0660030745687196,
-0.985429844592535));
#37961=CARTESIAN_POINT('Ctrl Pts',(0.157471990835318,0.12253361091382,-0.974310198850936));
#37962=CARTESIAN_POINT('Ctrl Pts',(-0.0175707445788509,0.198809961672541,
-0.963190553109335));
#37963=CARTESIAN_POINT('Ctrl Pts',(-0.17665014620923,0.0929356538694735,
-0.952070907367737));
#37964=CARTESIAN_POINT('Ctrl Pts',(-0.1738129205952,-0.0980847992252637,
-0.940951261626134));
#37965=CARTESIAN_POINT('Ctrl Pts',(-0.0117662937611897,-0.19924099893454,
-0.929831615884536));
#37966=CARTESIAN_POINT('Ctrl Pts',(0.161080028803121,-0.117853348200155,
-0.918711970142934));
#37967=CARTESIAN_POINT('Ctrl Pts',(0.186335434701197,0.0715107835544593,
-0.907592324401336));
#37968=CARTESIAN_POINT('Ctrl Pts',(0.0408766512511551,0.195357182547014,
-0.896472678659735));
#37969=CARTESIAN_POINT('Ctrl Pts',(-0.142035928933471,0.140218302045289,
-0.885353032918135));
#37970=CARTESIAN_POINT('Ctrl Pts',(-0.194814445340139,-0.0433878395750506,
-0.874233387176535));
#37971=CARTESIAN_POINT('Ctrl Pts',(-0.0691057534074772,-0.1872422783597,
-0.863113741434934));
#37972=CARTESIAN_POINT('Ctrl Pts',(0.119917680411353,-0.1595463053667,-0.851994095693335));
#37973=CARTESIAN_POINT('Ctrl Pts',(0.199072941868794,0.014325163437664,
-0.840874449951735));
#37974=CARTESIAN_POINT('Ctrl Pts',(0.0958387173699031,0.175071993284764,
-0.829754804210135));
#37975=CARTESIAN_POINT('Ctrl Pts',(-0.0952025028943739,0.175418768523093,
-0.818635158468535));
#37976=CARTESIAN_POINT('Ctrl Pts',(-0.199019651887221,0.0150477767656126,
-0.807515512726934));
#37977=CARTESIAN_POINT('Ctrl Pts',(-0.120496042611065,-0.159109910383761,
-0.796395866985335));
#37978=CARTESIAN_POINT('Ctrl Pts',(0.068425425567148,-0.187491921353828,
-0.785276221243733));
#37979=CARTESIAN_POINT('Ctrl Pts',(0.194655868635495,-0.0440948048366693,
-0.774156575502135));
#37980=CARTESIAN_POINT('Ctrl Pts',(0.142543615107852,0.139701743592238,
-0.763036929760534));
#37981=CARTESIAN_POINT('Ctrl Pts',(-0.0401663617616404,0.195504277869735,
-0.751917284018934));
#37982=CARTESIAN_POINT('Ctrl Pts',(-0.18607612530664,0.0721868050513496,
-0.740797638277334));
#37983=CARTESIAN_POINT('Ctrl Pts',(-0.16150390664979,-0.117267844792243,
-0.729677992535734));
#37984=CARTESIAN_POINT('Ctrl Pts',(0.0110373552267338,-0.199282302422261,
-0.718558346794134));
#37985=CARTESIAN_POINT('Ctrl Pts',(0.173466249299268,-0.0987153464152002,
-0.707438701052533));
#37986=CARTESIAN_POINT('Ctrl Pts',(0.176966263984219,0.0922940988513697,
-0.696319055310934));
#37987=CARTESIAN_POINT('Ctrl Pts',(0.0183307038740293,0.198744168628912,
-0.685199409569334));
#37988=CARTESIAN_POINT('Ctrl Pts',(-0.157099352199452,0.123105860163347,
-0.674079763827732));
#37989=CARTESIAN_POINT('Ctrl Pts',(-0.188595795221582,-0.0653213999683454,
-0.662960118086134));
#37990=CARTESIAN_POINT('Ctrl Pts',(-0.0473017471663473,-0.193901531669128,
-0.651840472344532));
#37991=CARTESIAN_POINT('Ctrl Pts',(0.137329916722456,-0.144830084035059,
-0.640720826602934));
#37992=CARTESIAN_POINT('Ctrl Pts',(0.19614062197592,0.0369339366929576,
-0.629601180861333));
#37993=CARTESIAN_POINT('Ctrl Pts',(0.0752483049484038,0.184859275858851,
-0.618481535119733));
#37994=CARTESIAN_POINT('Ctrl Pts',(-0.114586119453036,0.16341750364439,
-0.607361889378132));
#37995=CARTESIAN_POINT('Ctrl Pts',(-0.199437334514005,-0.00774653926841995,
-0.596242243636534));
#37996=CARTESIAN_POINT('Ctrl Pts',(-0.101565096336734,-0.171813243013414,
-0.585122597894932));
#37997=CARTESIAN_POINT('Ctrl Pts',(0.089360557222013,-0.178465543121493,
-0.574002952153333));
#37998=CARTESIAN_POINT('Ctrl Pts',(0.198414530943696,-0.0216086366778103,
-0.562883306411733));
#37999=CARTESIAN_POINT('Ctrl Pts',(0.125682138762467,0.155045990805214,
-0.551763660670133));
#38000=CARTESIAN_POINT('Ctrl Pts',(-0.062199578197878,0.189648284307254,
-0.540644014928533));
#38001=CARTESIAN_POINT('Ctrl Pts',(-0.193094363669353,0.0504958016849643,
-0.529524369186932));
#38002=CARTESIAN_POINT('Ctrl Pts',(-0.147077092947998,-0.134920672984703,
-0.518404723445333));
#38003=CARTESIAN_POINT('Ctrl Pts',(0.033691448798796,-0.196723525655976,
-0.507285077703731));
#38004=CARTESIAN_POINT('Ctrl Pts',(0.1835920596032,-0.0782893027132967,
-0.496165431962133));
#38005=CARTESIAN_POINT('Ctrl Pts',(0.165286575999301,0.111873174010154,
-0.485045786220532));
#38006=CARTESIAN_POINT('Ctrl Pts',(-0.0044536127168597,0.199538027960706,
-0.473926140478932));
#38007=CARTESIAN_POINT('Ctrl Pts',(-0.170113424521682,0.104387173858599,
-0.462806494737332));
#38008=CARTESIAN_POINT('Ctrl Pts',(-0.179916197590418,-0.0864026684384514,
-0.451686848995732));
#38009=CARTESIAN_POINT('Ctrl Pts',(-0.0248806819941409,-0.1980308332866,
-0.440567203254132));
#38010=CARTESIAN_POINT('Ctrl Pts',(0.152950385618357,-0.12822417403858,
-0.429447557512532));
#38011=CARTESIAN_POINT('Ctrl Pts',(0.19064910187147,0.0590608095464339,
-0.418327911770931));
#38012=CARTESIAN_POINT('Ctrl Pts',(0.0536760981299502,0.192234585229143,
-0.407208266029333));
#38013=CARTESIAN_POINT('Ctrl Pts',(-0.13247466879498,0.149284029274227,
-0.396088620287731));
#38014=CARTESIAN_POINT('Ctrl Pts',(-0.197252830095204,-0.0304397813412365,
-0.384968974546132));
#38015=CARTESIAN_POINT('Ctrl Pts',(-0.0813089697949813,-0.182274821902383,
-0.373849328804531));
#38016=CARTESIAN_POINT('Ctrl Pts',(0.109129747631262,-0.167110614416551,
-0.362729683062932));
#38017=CARTESIAN_POINT('Ctrl Pts',(0.199584355327704,0.00115947273534765,
-0.351610037321331));
#38018=CARTESIAN_POINT('Ctrl Pts',(0.107180810078425,0.168367256969862,
-0.340490391579731));
#38019=CARTESIAN_POINT('Ctrl Pts',(-0.0834212384069029,0.181317832139435,
-0.329370745838131));
#38020=CARTESIAN_POINT('Ctrl Pts',(-0.197593180198466,0.0281459483247914,
-0.318251100096531));
#38021=CARTESIAN_POINT('Ctrl Pts',(-0.130731273392021,-0.15081310760612,
-0.307131454354931));
#38022=CARTESIAN_POINT('Ctrl Pts',(0.0559059492071229,-0.191597975236089,
-0.296011808613331));
#38023=CARTESIAN_POINT('Ctrl Pts',(0.191322430593934,-0.0568417699887867,
-0.284892162871731));
#38024=CARTESIAN_POINT('Ctrl Pts',(0.151450291730699,0.129992570571571,
-0.273772517130131));
#38025=CARTESIAN_POINT('Ctrl Pts',(-0.0271798203035159,0.19772839111678,
-0.262652871388531));
#38026=CARTESIAN_POINT('Ctrl Pts',(-0.180907921584439,0.0843064833844511,
-0.251533225646931));
#38027=CARTESIAN_POINT('Ctrl Pts',(-0.168889122045176,-0.106356587653718,
-0.240413579905331));
#38028=CARTESIAN_POINT('Ctrl Pts',(-0.00213498291551102,-0.199576304251475,
-0.229293934163731));
#38029=CARTESIAN_POINT('Ctrl Pts',(0.16657521566113,-0.109945243349912,
-0.218174288422131));
#38030=CARTESIAN_POINT('Ctrl Pts',(0.182670065750174,0.0804170785083747,
-0.20705464268053));
#38031=CARTESIAN_POINT('Ctrl Pts',(0.0314035443582194,0.19710169270962,
-0.19593499693893));
#38032=CARTESIAN_POINT('Ctrl Pts',(-0.148634735933524,0.133202750335231,
-0.18481535119733));
#38033=CARTESIAN_POINT('Ctrl Pts',(-0.192494651883585,-0.0527358502702753,
-0.17369570545573));
#38034=CARTESIAN_POINT('Ctrl Pts',(-0.0599919432941398,-0.190358160633059,
-0.16257605971413));
#38035=CARTESIAN_POINT('Ctrl Pts',(0.127475032783534,-0.153575266591495,
-0.15145641397253));
#38036=CARTESIAN_POINT('Ctrl Pts',(0.198150120668658,0.023912409129983,
-0.14033676823093));
#38037=CARTESIAN_POINT('Ctrl Pts',(0.0872809477146552,0.179491816318678,
-0.12921712248933));
#38038=CARTESIAN_POINT('Ctrl Pts',(-0.103554299087435,0.170621451982705,
-0.11809747674773));
#38039=CARTESIAN_POINT('Ctrl Pts',(-0.199514163646704,0.00542916575673231,
-0.10697783100613));
#38040=CARTESIAN_POINT('Ctrl Pts',(-0.112679174471304,-0.164738377528375,
-0.09585818526453));
#38041=CARTESIAN_POINT('Ctrl Pts',(0.0773899674941174,-0.183971408977363,
-0.0847385395229295));
#38042=CARTESIAN_POINT('Ctrl Pts',(0.196558484758314,-0.0346547172938525,
-0.0736188937813297));
#38043=CARTESIAN_POINT('Ctrl Pts',(0.135634160884303,0.146419929403477,
-0.0624992480397295));
#38044=CARTESIAN_POINT('Ctrl Pts',(-0.0495441958477198,0.193331145609538,
-0.0513796022981294));
#38045=CARTESIAN_POINT('Ctrl Pts',(-0.189355714081398,0.0631405057044453,
-0.0402599565565294));
#38046=CARTESIAN_POINT('Ctrl Pts',(-0.155632314932806,-0.124950848232207,
-0.0291403108149293));
#38047=CARTESIAN_POINT('Ctrl Pts',(0.0205886678373547,-0.198464154088089,
-0.0180206650733292));
#38048=CARTESIAN_POINT('Ctrl Pts',(0.178122917610402,-0.09033586191714,
-0.00690101933172914));
#38049=CARTESIAN_POINT('Ctrl Pts',(0.172113458958819,0.100939087356816,
0.00421862640987089));
#38050=CARTESIAN_POINT('Ctrl Pts',(0.0634944322694335,0.166217620505429,
0.0116317235709377));
#38051=CARTESIAN_POINT('Ctrl Pts',(0.00737739821677849,0.168672073681435,
0.015338272151471));
#38052=CARTESIAN_POINT('Ctrl Pts',(-0.107438039834496,-0.112484977203719,
-1.));
#38053=CARTESIAN_POINT('Ctrl Pts',(-0.070014397862351,-0.148229508046032,
-0.996293451419467));
#38054=CARTESIAN_POINT('Ctrl Pts',(0.0426645675892999,-0.178810969987729,
-0.988880354258401));
#38055=CARTESIAN_POINT('Ctrl Pts',(0.173668580798161,-0.0608101377048221,
-0.977760708516799));
#38056=CARTESIAN_POINT('Ctrl Pts',(0.145082536077593,0.112893009936692,
-0.9666410627752));
#38057=CARTESIAN_POINT('Ctrl Pts',(-0.016188327655916,0.183168151262569,
-0.9555214170336));
#38058=CARTESIAN_POINT('Ctrl Pts',(-0.162751807953678,0.0856237371731279,
-0.944401771292001));
#38059=CARTESIAN_POINT('Ctrl Pts',(-0.160137807296644,-0.0903677622082326,
-0.933282125550398));
#38060=CARTESIAN_POINT('Ctrl Pts',(-0.0108405547554956,-0.183565275721231,
-0.922162479808802));
#38061=CARTESIAN_POINT('Ctrl Pts',(0.148406703733419,-0.108580977171968,
-0.911042834067198));
#38062=CARTESIAN_POINT('Ctrl Pts',(0.171675085100322,0.0658845155887245,
-0.899923188325601));
#38063=CARTESIAN_POINT('Ctrl Pts',(0.037660590930604,0.179987027118587,
-0.888803542583998));
#38064=CARTESIAN_POINT('Ctrl Pts',(-0.130860940250355,0.129186319149918,
-0.8776838968424));
#38065=CARTESIAN_POINT('Ctrl Pts',(-0.179486990953555,-0.0399742059974294,
-0.866564251100799));
#38066=CARTESIAN_POINT('Ctrl Pts',(-0.0636687064710734,-0.17251058084216,
-0.8554446053592));
#38067=CARTESIAN_POINT('Ctrl Pts',(0.110482893512257,-0.146993649357098,
-0.844324959617598));
#38068=CARTESIAN_POINT('Ctrl Pts',(0.18341044091426,0.0131980997397562,
-0.833205313875999));
#38069=CARTESIAN_POINT('Ctrl Pts',(0.0882983957762384,0.161297819676871,
-0.822085668134399));
#38070=CARTESIAN_POINT('Ctrl Pts',(-0.0877122368719845,0.161617311611651,
-0.810966022392799));
#38071=CARTESIAN_POINT('Ctrl Pts',(-0.183361343639036,0.0138638598769447,
-0.799846376651199));
#38072=CARTESIAN_POINT('Ctrl Pts',(-0.111015751795564,-0.146591588707962,
-0.7887267309096));
#38073=CARTESIAN_POINT('Ctrl Pts',(0.0630419049178878,-0.172740582625397,
-0.777607085167998));
#38074=CARTESIAN_POINT('Ctrl Pts',(0.179340890619455,-0.0406255492142766,
-0.766487439426399));
#38075=CARTESIAN_POINT('Ctrl Pts',(0.131328683099859,0.128710402067756,
-0.755367793684797));
#38076=CARTESIAN_POINT('Ctrl Pts',(-0.037006185026792,0.180122549393705,
-0.7442481479432));
#38077=CARTESIAN_POINT('Ctrl Pts',(-0.171436177441942,0.0665073496095001,
-0.733128502201597));
#38078=CARTESIAN_POINT('Ctrl Pts',(-0.148797232059476,-0.108041539530703,
-0.722008856459999));
#38079=CARTESIAN_POINT('Ctrl Pts',(0.0101689670613149,-0.183603329566334,
-0.710889210718397));
#38080=CARTESIAN_POINT('Ctrl Pts',(0.159818411126364,-0.0909486997130359,
-0.6997695649768));
#38081=CARTESIAN_POINT('Ctrl Pts',(0.163043054468382,0.0850326579052167,
-0.688649919235197));
#38082=CARTESIAN_POINT('Ctrl Pts',(0.0168884954843339,0.183107534631158,
-0.677530273493599));
#38083=CARTESIAN_POINT('Ctrl Pts',(-0.144739215604886,0.113420236219596,
-0.666410627751997));
#38084=CARTESIAN_POINT('Ctrl Pts',(-0.173757606792006,-0.0601820953508962,
-0.655290982010399));
#38085=CARTESIAN_POINT('Ctrl Pts',(-0.0435801783122908,-0.178645902770777,
-0.644171336268797));
#38086=CARTESIAN_POINT('Ctrl Pts',(0.126525183886544,-0.133435259062113,
-0.633051690527199));
#38087=CARTESIAN_POINT('Ctrl Pts',(0.180708827729641,0.0340280781002357,
-0.621932044785597));
#38088=CARTESIAN_POINT('Ctrl Pts',(0.0693279792777336,0.170315066297202,
-0.610812399043998));
#38089=CARTESIAN_POINT('Ctrl Pts',(-0.105570804822823,0.150560272607413,
-0.599692753302398));
#38090=CARTESIAN_POINT('Ctrl Pts',(-0.18374616416774,-0.00713706327662168,
-0.588573107560797));
#38091=CARTESIAN_POINT('Ctrl Pts',(-0.0935742393001708,-0.15829545874079,
-0.577453461819198));
#38092=CARTESIAN_POINT('Ctrl Pts',(0.0823299191069159,-0.164424374526445,
-0.566333816077597));
#38093=CARTESIAN_POINT('Ctrl Pts',(0.182803831914859,-0.0199085297249743,
-0.555214170335998));
#38094=CARTESIAN_POINT('Ctrl Pts',(0.115793820441273,0.142847406928437,
-0.544094524594397));
#38095=CARTESIAN_POINT('Ctrl Pts',(-0.057305889765134,0.174727288987128,
-0.532974878852797));
#38096=CARTESIAN_POINT('Ctrl Pts',(-0.177902240486286,0.0465229335760867,
-0.521855233111197));
#38097=CARTESIAN_POINT('Ctrl Pts',(-0.135505479613391,-0.124305492691633,
-0.510735587369597));
#38098=CARTESIAN_POINT('Ctrl Pts',(0.0310407000630972,-0.181245870182351,
-0.499615941627997));
#38099=CARTESIAN_POINT('Ctrl Pts',(0.169147551063838,-0.0721297198640855,
-0.488496295886397));
#38100=CARTESIAN_POINT('Ctrl Pts',(0.152282291589484,0.103071306321499,
-0.477376650144796));
#38101=CARTESIAN_POINT('Ctrl Pts',(-0.00410321495424111,0.183838935336354,
-0.466257004403197));
#38102=CARTESIAN_POINT('Ctrl Pts',(-0.156729377202455,0.096174283674461,
-0.455137358661596));
#38103=CARTESIAN_POINT('Ctrl Pts',(-0.165760895568743,-0.0796047487202445,
-0.444017712919997));
#38104=CARTESIAN_POINT('Ctrl Pts',(-0.0229231396891714,-0.182450322513706,
-0.432898067178396));
#38105=CARTESIAN_POINT('Ctrl Pts',(0.140916678082541,-0.118135855508594,
-0.421778421436797));
#38106=CARTESIAN_POINT('Ctrl Pts',(0.175649365031236,0.0544140706314786,
-0.410658775695196));
#38107=CARTESIAN_POINT('Ctrl Pts',(0.0494530132129136,0.177110107003317,
-0.399539129953596));
#38108=CARTESIAN_POINT('Ctrl Pts',(-0.122051933254053,0.137538780376738,
-0.388419484211996));
#38109=CARTESIAN_POINT('Ctrl Pts',(-0.181733530432234,-0.0280448646848738,
-0.377299838470396));
#38110=CARTESIAN_POINT('Ctrl Pts',(-0.0749118080055823,-0.167933949932374,
-0.366180192728796));
#38111=CARTESIAN_POINT('Ctrl Pts',(0.100543725038754,-0.153962819777854,
-0.355060546987196));
#38112=CARTESIAN_POINT('Ctrl Pts',(0.183881617795998,0.00106824867117576,
-0.343940901245595));
#38113=CARTESIAN_POINT('Ctrl Pts',(0.0987481244286207,0.155120593218137,
-0.332821255503996));
#38114=CARTESIAN_POINT('Ctrl Pts',(-0.0768578892449788,0.167052253441001,
-0.321701609762395));
#38115=CARTESIAN_POINT('Ctrl Pts',(-0.182047102743562,0.025931504019276,
-0.310581964020796));
#38116=CARTESIAN_POINT('Ctrl Pts',(-0.120445703313694,-0.138947555112332,
-0.299462318279195));
#38117=CARTESIAN_POINT('Ctrl Pts',(0.0515074258588442,-0.176523583699745,
-0.288342672537596));
#38118=CARTESIAN_POINT('Ctrl Pts',(0.176269718137531,-0.0523696188850282,
-0.277223026795995));
#38119=CARTESIAN_POINT('Ctrl Pts',(0.139534607376368,0.119765119560166,
-0.266103381054396));
#38120=CARTESIAN_POINT('Ctrl Pts',(-0.0250413882421251,0.182171675645894,
-0.254983735312795));
#38121=CARTESIAN_POINT('Ctrl Pts',(-0.166674593499267,0.0776734856295233,
-0.243864089571196));
#38122=CARTESIAN_POINT('Ctrl Pts',(-0.155601399412401,-0.0979887495135398,
-0.232744443829595));
#38123=CARTESIAN_POINT('Ctrl Pts',(-0.00196700844525682,-0.183874200155875,
-0.221624798087995));
#38124=CARTESIAN_POINT('Ctrl Pts',(0.153469544695492,-0.101295059840545,
-0.210505152346395));
#38125=CARTESIAN_POINT('Ctrl Pts',(0.168298097102307,0.074090088224943,
-0.199385506604795));
#38126=CARTESIAN_POINT('Ctrl Pts',(0.0289328015296395,0.181594284112427,
-0.188265860863195));
#38127=CARTESIAN_POINT('Ctrl Pts',(-0.136940571615754,0.122722731379931,
-0.177146215121595));
#38128=CARTESIAN_POINT('Ctrl Pts',(-0.177349712342497,-0.0485867414188046,
-0.166026569379995));
#38129=CARTESIAN_POINT('Ctrl Pts',(-0.0552719453863964,-0.175381314233795,
-0.154906923638395));
#38130=CARTESIAN_POINT('Ctrl Pts',(0.117445654587239,-0.141492395172598,
-0.143787277896795));
#38131=CARTESIAN_POINT('Ctrl Pts',(0.182560224698972,0.0220310478193626,
-0.132667632155195));
#38132=CARTESIAN_POINT('Ctrl Pts',(0.0804139274452977,0.165369903425689,
-0.121547986413595));
#38133=CARTESIAN_POINT('Ctrl Pts',(-0.0954069371552854,0.157197434487125,
-0.110428340671994));
#38134=CARTESIAN_POINT('Ctrl Pts',(-0.183816948599673,0.00500201421594969,
-0.0993086949303943));
#38135=CARTESIAN_POINT('Ctrl Pts',(-0.103813892926028,-0.151777223837348,
-0.0881890491887944));
#38136=CARTESIAN_POINT('Ctrl Pts',(0.0713011418186189,-0.169497054292766,
-0.0770694034471942));
#38137=CARTESIAN_POINT('Ctrl Pts',(0.181093814239817,-0.0319281812935353,
-0.065949757705594));
#38138=CARTESIAN_POINT('Ctrl Pts',(0.124962845363592,0.134900019854162,
-0.0548301119639941));
#38139=CARTESIAN_POINT('Ctrl Pts',(-0.045646197418241,0.178120393087247,
-0.0437104662223939));
#38140=CARTESIAN_POINT('Ctrl Pts',(-0.174457737366406,0.0581727877334231,
-0.0325908204807939));
#38141=CARTESIAN_POINT('Ctrl Pts',(-0.143387600717461,-0.115120065799724,
-0.0214711747391938));
#38142=CARTESIAN_POINT('Ctrl Pts',(0.0189688091733509,-0.182849550849372,
-0.0103515289975937));
#38143=CARTESIAN_POINT('Ctrl Pts',(0.164108705829999,-0.0832284895629474,
0.00076811674400635));
#38144=CARTESIAN_POINT('Ctrl Pts',(0.158572054537281,0.0929974829517444,
0.0118877624856064));
#38145=CARTESIAN_POINT('Ctrl Pts',(0.0584988683485304,0.153140084124104,
0.0193008596466731));
#38146=CARTESIAN_POINT('Ctrl Pts',(0.00679696520801413,0.155401427805413,
0.0230074082272065));
#38147=CARTESIAN_POINT('',(0.00853826423430722,0.195213365433479,0.));
#38148=CARTESIAN_POINT('Ctrl Pts',(0.133822070517493,-0.0798006560480865,
1.04083408558608E-17));
#38149=CARTESIAN_POINT('Ctrl Pts',(0.136054490212563,-0.0769648097335247,
3.49555778604013E-18));
#38150=CARTESIAN_POINT('Ctrl Pts',(0.13817734199536,-0.0740511128945859,
1.83743250757632E-16));
#38151=CARTESIAN_POINT('Ctrl Pts',(0.14018477846174,-0.0710636564573235,
1.94289029309402E-16));
#38152=CARTESIAN_POINT('Ctrl Pts',(0.145087642260683,-0.063767240225737,
2.23391728783535E-16));
#38153=CARTESIAN_POINT('Ctrl Pts',(0.149303339241034,-0.0560321219577389,
1.56818419132082E-16));
#38154=CARTESIAN_POINT('Ctrl Pts',(0.152847589720857,-0.0479613923182007,
1.2490009027033E-16));
#38155=CARTESIAN_POINT('Ctrl Pts',(0.15455977808461,-0.0440625117355556,
1.09480697205803E-16));
#38156=CARTESIAN_POINT('Ctrl Pts',(0.156114761257445,-0.0400845646834566,
-1.25648886706941E-16));
#38157=CARTESIAN_POINT('Ctrl Pts',(0.157508730347866,-0.0360533266198954,
-6.93889390390723E-17));
#38158=CARTESIAN_POINT('Ctrl Pts',(0.160055180865878,-0.0286892119306038,
3.3384625932115E-17));
#38159=CARTESIAN_POINT('Ctrl Pts',(0.162070216310737,-0.0211365082118436,
8.06994689406633E-17));
#38160=CARTESIAN_POINT('Ctrl Pts',(0.163561952707671,-0.0134617511743051,
6.93889390390723E-17));
#38161=CARTESIAN_POINT('Ctrl Pts',(0.164339267575536,-0.00946258432097103,
6.34952415506897E-17));
#38162=CARTESIAN_POINT('Ctrl Pts',(0.164974517612341,-0.00542855824006687,
1.57353126539468E-16));
#38163=CARTESIAN_POINT('Ctrl Pts',(0.165467142704647,-0.00137336699737669,
1.35308431126191E-16));
#38164=CARTESIAN_POINT('Ctrl Pts',(0.166873643263939,0.0102046643290036,
7.23683232988437E-17));
#38165=CARTESIAN_POINT('Ctrl Pts',(0.167113195337005,0.0218827002968643,
1.56622012929874E-16));
#38166=CARTESIAN_POINT('Ctrl Pts',(0.166211473778159,0.0334541513985393,
2.42861286636753E-16));
#38167=CARTESIAN_POINT('Ctrl Pts',(0.165524281373494,0.0422726311498785,
3.08583319445951E-16));
#38168=CARTESIAN_POINT('Ctrl Pts',(0.164173427571641,0.0510302884111691,
1.90686017996932E-16));
#38169=CARTESIAN_POINT('Ctrl Pts',(0.162151293669402,0.0596413236714313,
2.39391839684799E-16));
#38170=CARTESIAN_POINT('Ctrl Pts',(0.161342806590566,0.0630841771519127,
2.58865341145375E-16));
#38171=CARTESIAN_POINT('Ctrl Pts',(0.160426561788868,0.0665033606500684,
2.97312651021588E-16));
#38172=CARTESIAN_POINT('Ctrl Pts',(0.159406336715296,0.0698797924692321,
2.84494650060196E-16));
#38173=CARTESIAN_POINT('Ctrl Pts',(0.157424304970836,0.0764393205791983,
2.59592610829727E-16));
#38174=CARTESIAN_POINT('Ctrl Pts',(0.155047364014314,0.0828505294531396,
1.84123669457675E-18));
#38175=CARTESIAN_POINT('Ctrl Pts',(0.152277239552743,0.0890746728807261,
3.46944695195361E-18));
#38176=CARTESIAN_POINT('Ctrl Pts',(0.149146033051636,0.0961101251265181,
5.25576150690907E-18));
#38177=CARTESIAN_POINT('Ctrl Pts',(0.145512730626329,0.102906823780167,
-5.8747241662667E-17));
#38178=CARTESIAN_POINT('Ctrl Pts',(0.141425681028324,0.109443008062494,
-1.21430643318376E-16));
#38179=CARTESIAN_POINT('Ctrl Pts',(0.138942944415873,0.113413506495247,
-1.59508570329487E-16));
#38180=CARTESIAN_POINT('Ctrl Pts',(0.13629256386344,0.117287832803984,1.53692496207997E-16));
#38181=CARTESIAN_POINT('Ctrl Pts',(0.133483702160606,0.121060495400109,
1.6306400674182E-16));
#38182=CARTESIAN_POINT('Ctrl Pts',(0.131345168294252,0.123932821481525,
1.70199029671303E-16));
#38183=CARTESIAN_POINT('Ctrl Pts',(0.129114839715568,0.126745619606885,
5.90473990481052E-17));
#38184=CARTESIAN_POINT('Ctrl Pts',(0.126805988740716,0.129486179768006,
4.5102810375397E-17));
#38185=CARTESIAN_POINT('Ctrl Pts',(0.11940504484662,0.138270952891856,4.03901906608835E-19));
#38186=CARTESIAN_POINT('Ctrl Pts',(0.111179428463956,0.146343614865738,
2.51922702503768E-18));
#38187=CARTESIAN_POINT('Ctrl Pts',(0.102279336934698,0.153635544773705,
-1.4658413372004E-16));
#38188=CARTESIAN_POINT('Ctrl Pts',(0.0968240568380823,0.158105107807083,
-2.37976519240706E-16));
#38189=CARTESIAN_POINT('Ctrl Pts',(0.0911145357147371,0.162281120633163,
-2.06184360493938E-16));
#38190=CARTESIAN_POINT('Ctrl Pts',(0.0851790897705271,0.166143964756861,
-1.63931368479808E-16));
#38191=CARTESIAN_POINT('Ctrl Pts',(0.0807002479834999,0.169058837175987,
-1.32047586193085E-16));
#38192=CARTESIAN_POINT('Ctrl Pts',(0.0760870922293099,0.171797833033742,
-1.31664209440999E-18));
#38193=CARTESIAN_POINT('Ctrl Pts',(0.0713813828666237,0.174335786156758,
-3.46944695195361E-18));
#38194=CARTESIAN_POINT('Ctrl Pts',(0.060093655680461,0.180423650972855,
-8.63344499009989E-18));
#38195=CARTESIAN_POINT('Ctrl Pts',(0.0482526397033331,0.185375716453591,
2.38150771112053E-17));
#38196=CARTESIAN_POINT('Ctrl Pts',(0.0360316133450007,0.189089719698973,
2.86229373536173E-17));
#38197=CARTESIAN_POINT('Ctrl Pts',(0.0270536221211358,0.191818155721019,
3.21549587891586E-17));
#38198=CARTESIAN_POINT('Ctrl Pts',(0.0178694527935419,0.19387797767402,
2.08963768332319E-17));
#38199=CARTESIAN_POINT('Ctrl Pts',(0.00853826423430726,0.195213365433479,
-1.73472347597681E-18));
#38200=CARTESIAN_POINT('Ctrl Pts',(0.00853826423430726,0.195213365433479,
-1.73472347597681E-18));
#38201=CARTESIAN_POINT('Ctrl Pts',(0.0734855601112398,0.192372693268079,
-0.00370654858053334));
#38202=CARTESIAN_POINT('Ctrl Pts',(0.136340913956568,0.154597494717519,
-0.00741309716106669));
#38203=CARTESIAN_POINT('Ctrl Pts',(0.168927769774117,0.0988144116434918,
-0.0111196457416));
#38204=CARTESIAN_POINT('Ctrl Pts',(0.201514625591668,0.0430313285694631,
-0.0148261943221335));
#38205=CARTESIAN_POINT('Ctrl Pts',(0.203832983381438,-0.0307596390280334,
-0.0185327429026669));
#38206=CARTESIAN_POINT('Ctrl Pts',(0.174605002942014,-0.0885122484834479,
-0.0222392914832004));
#38207=CARTESIAN_POINT('Ctrl Pts',(0.145377022502591,-0.14626485793886,
-0.0259458400637337));
#38208=CARTESIAN_POINT('Ctrl Pts',(0.0846027038339767,-0.187979109252192,
-0.0296523886442669));
#38209=CARTESIAN_POINT('Ctrl Pts',(0.0202238564115267,-0.194656076997466,
-0.0333589372248002));
#38210=CARTESIAN_POINT('Ctrl Pts',(-0.0441549910109242,-0.201333044742741,
-0.0370654858053336));
#38211=CARTESIAN_POINT('Ctrl Pts',(-0.112138367187211,-0.172972728919958,
-0.0407720343858669));
#38212=CARTESIAN_POINT('Ctrl Pts',(-0.152635042633335,-0.122511178551289,
-0.0444785829664003));
#38213=CARTESIAN_POINT('Ctrl Pts',(-0.180074773643688,-0.0883194491505946,
-0.0469900655734589));
#38214=CARTESIAN_POINT('Ctrl Pts',(-0.194894963322837,-0.0439807237331546,
-0.0495015481805176));
#38215=CARTESIAN_POINT('Ctrl Pts',(-0.195233177397639,0.000155192514023357,
-0.0520130307875762));
#38216=CARTESIAN_POINT('Origin',(0.,0.,-0.56));
#38217=CARTESIAN_POINT('Origin',(0.,0.,0.));
#38218=CARTESIAN_POINT('Origin',(0.,0.,0.67));
#38219=CARTESIAN_POINT('',(0.,0.,0.64));
#38220=CARTESIAN_POINT('',(-0.2,-2.44929359829471E-17,0.7));
#38221=CARTESIAN_POINT('',(-0.1,-1.22464679914735E-17,0.67));
#38222=CARTESIAN_POINT('Origin',(0.,0.,0.7));
#38223=CARTESIAN_POINT('Origin',(0.545748091853324,-0.146232760482925,0.06));
#38224=CARTESIAN_POINT('',(0.574066611494015,-0.174492193429331,0.06));
#38225=CARTESIAN_POINT('',(0.574066611494015,-0.174492193429331,0.59));
#38226=CARTESIAN_POINT('',(0.574066611494015,-0.174492193429331,0.325));
#38227=CARTESIAN_POINT('',(0.545748091853324,-0.146232760482925,0.06));
#38228=CARTESIAN_POINT('',(0.545748091853324,-0.146232760482925,0.06));
#38229=CARTESIAN_POINT('',(0.545748091853324,-0.146232760482925,0.59));
#38230=CARTESIAN_POINT('',(0.545748091853324,-0.146232760482925,0.06));
#38231=CARTESIAN_POINT('',(0.545748091853324,-0.146232760482925,0.59));
#38232=CARTESIAN_POINT('Origin',(0.581970310339164,-0.155938474674269,0.59));
#38233=CARTESIAN_POINT('',(0.584402365732934,-0.13591863347514,0.59));
#38234=CARTESIAN_POINT('Origin',(0.,0.,0.59));
#38235=CARTESIAN_POINT('',(0.629372708972173,-0.123919188518606,0.59));
#38236=CARTESIAN_POINT('Origin',(0.629372708972173,-0.123919188518606,0.06));
#38237=CARTESIAN_POINT('',(0.584402365732934,-0.13591863347514,0.06));
#38238=CARTESIAN_POINT('',(0.584402365732934,-0.13591863347514,0.325));
#38239=CARTESIAN_POINT('',(0.629372708972173,-0.123919188518606,0.06));
#38240=CARTESIAN_POINT('Origin',(0.581970310339164,-0.155938474674269,0.06));
#38241=CARTESIAN_POINT('Origin',(0.,0.,0.06));
#38242=CARTESIAN_POINT('Origin',(0.489304353138208,-0.2825,0.06));
#38243=CARTESIAN_POINT('',(0.509343863171099,-0.317125888331339,0.06));
#38244=CARTESIAN_POINT('',(0.509343863171099,-0.317125888331339,0.59));
#38245=CARTESIAN_POINT('',(0.509343863171099,-0.317125888331339,0.325));
#38246=CARTESIAN_POINT('',(0.489304353138208,-0.2825,0.06));
#38247=CARTESIAN_POINT('',(0.489304353138208,-0.2825,0.06));
#38248=CARTESIAN_POINT('',(0.489304353138208,-0.2825,0.59));
#38249=CARTESIAN_POINT('',(0.489304353138208,-0.2825,0.06));
#38250=CARTESIAN_POINT('',(0.489304353138208,-0.2825,0.59));
#38251=CARTESIAN_POINT('Origin',(0.521780305780124,-0.30125,0.59));
#38252=CARTESIAN_POINT('',(0.529311007078196,-0.282541780602208,0.59));
#38253=CARTESIAN_POINT('Origin',(0.,0.,0.59));
#38254=CARTESIAN_POINT('',(0.57585470791547,-0.28259038811267,0.59));
#38255=CARTESIAN_POINT('Origin',(0.57585470791547,-0.28259038811267,0.06));
#38256=CARTESIAN_POINT('',(0.529311007078196,-0.282541780602208,0.06));
#38257=CARTESIAN_POINT('',(0.529311007078196,-0.282541780602208,0.325));
#38258=CARTESIAN_POINT('',(0.57585470791547,-0.28259038811267,0.06));
#38259=CARTESIAN_POINT('Origin',(0.521780305780124,-0.30125,0.06));
#38260=CARTESIAN_POINT('Origin',(0.,0.,0.06));
#38261=CARTESIAN_POINT('Origin',(0.399515331370399,-0.3995153313704,0.06));
#38262=CARTESIAN_POINT('',(0.409910172303604,-0.438147978018876,0.06));
#38263=CARTESIAN_POINT('',(0.409910172303604,-0.438147978018876,0.59));
#38264=CARTESIAN_POINT('',(0.409910172303604,-0.438147978018876,0.325));
#38265=CARTESIAN_POINT('',(0.399515331370399,-0.3995153313704,0.06));
#38266=CARTESIAN_POINT('',(0.399515331370399,-0.3995153313704,0.06));
#38267=CARTESIAN_POINT('',(0.399515331370399,-0.3995153313704,0.59));
#38268=CARTESIAN_POINT('',(0.399515331370399,-0.3995153313704,0.06));
#38269=CARTESIAN_POINT('',(0.399515331370399,-0.3995153313704,0.59));
#38270=CARTESIAN_POINT('Origin',(0.426031835664895,-0.426031835664895,0.59));
#38271=CARTESIAN_POINT('',(0.438147978018876,-0.409910172303604,0.59));
#38272=CARTESIAN_POINT('Origin',(0.,0.,0.59));
#38273=CARTESIAN_POINT('',(0.483093160159229,-0.422003519759552,0.59));
#38274=CARTESIAN_POINT('Origin',(0.483093160159229,-0.422003519759552,0.06));
#38275=CARTESIAN_POINT('',(0.438147978018876,-0.409910172303604,0.06));
#38276=CARTESIAN_POINT('',(0.438147978018876,-0.409910172303604,0.325));
#38277=CARTESIAN_POINT('',(0.483093160159229,-0.422003519759552,0.06));
#38278=CARTESIAN_POINT('Origin',(0.426031835664895,-0.426031835664895,0.06));
#38279=CARTESIAN_POINT('Origin',(0.,0.,0.06));
#38280=CARTESIAN_POINT('Origin',(0.2825,-0.489304353138208,0.06));
#38281=CARTESIAN_POINT('',(0.282541780602207,-0.529311007078196,0.06));
#38282=CARTESIAN_POINT('',(0.282541780602207,-0.529311007078196,0.59));
#38283=CARTESIAN_POINT('',(0.282541780602207,-0.529311007078196,0.325));
#38284=CARTESIAN_POINT('',(0.2825,-0.489304353138208,0.06));
#38285=CARTESIAN_POINT('',(0.2825,-0.489304353138208,0.06));
#38286=CARTESIAN_POINT('',(0.2825,-0.489304353138208,0.59));
#38287=CARTESIAN_POINT('',(0.2825,-0.489304353138208,0.06));
#38288=CARTESIAN_POINT('',(0.2825,-0.489304353138208,0.59));
#38289=CARTESIAN_POINT('Origin',(0.30125,-0.521780305780125,0.59));
#38290=CARTESIAN_POINT('',(0.317125888331339,-0.509343863171099,0.59));
#38291=CARTESIAN_POINT('Origin',(0.,0.,0.59));
#38292=CARTESIAN_POINT('',(0.35740961188733,-0.532657808928611,0.59));
#38293=CARTESIAN_POINT('Origin',(0.35740961188733,-0.532657808928611,0.06));
#38294=CARTESIAN_POINT('',(0.317125888331339,-0.509343863171099,0.06));
#38295=CARTESIAN_POINT('',(0.317125888331338,-0.509343863171099,0.325));
#38296=CARTESIAN_POINT('',(0.35740961188733,-0.532657808928611,0.06));
#38297=CARTESIAN_POINT('Origin',(0.30125,-0.521780305780125,0.06));
#38298=CARTESIAN_POINT('Origin',(0.,0.,0.06));
#38299=CARTESIAN_POINT('Origin',(0.146232760482924,-0.545748091853324,0.06));
#38300=CARTESIAN_POINT('',(0.135918633475139,-0.584402365732935,0.06));
#38301=CARTESIAN_POINT('',(0.135918633475139,-0.584402365732935,0.59));
#38302=CARTESIAN_POINT('',(0.135918633475139,-0.584402365732935,0.325));
#38303=CARTESIAN_POINT('',(0.146232760482924,-0.545748091853324,0.06));
#38304=CARTESIAN_POINT('',(0.146232760482924,-0.545748091853324,0.06));
#38305=CARTESIAN_POINT('',(0.146232760482924,-0.545748091853324,0.59));
#38306=CARTESIAN_POINT('',(0.146232760482924,-0.545748091853324,0.06));
#38307=CARTESIAN_POINT('',(0.146232760482924,-0.545748091853324,0.59));
#38308=CARTESIAN_POINT('Origin',(0.155938474674268,-0.581970310339164,0.59));
#38309=CARTESIAN_POINT('',(0.17449219342933,-0.574066611494016,0.59));
#38310=CARTESIAN_POINT('Origin',(0.,0.,0.59));
#38311=CARTESIAN_POINT('',(0.207369189212621,-0.607012348677835,0.59));
#38312=CARTESIAN_POINT('Origin',(0.207369189212621,-0.607012348677835,0.06));
#38313=CARTESIAN_POINT('',(0.17449219342933,-0.574066611494016,0.06));
#38314=CARTESIAN_POINT('',(0.17449219342933,-0.574066611494016,0.325));
#38315=CARTESIAN_POINT('',(0.207369189212621,-0.607012348677835,0.06));
#38316=CARTESIAN_POINT('Origin',(0.155938474674268,-0.581970310339164,0.06));
#38317=CARTESIAN_POINT('Origin',(0.,0.,0.06));
#38318=CARTESIAN_POINT('Origin',(-1.11022302462516E-16,-0.565,0.06));
#38319=CARTESIAN_POINT('',(-0.0199671439070973,-0.599667668933546,0.06));
#38320=CARTESIAN_POINT('',(-0.0199671439070973,-0.599667668933546,0.59));
#38321=CARTESIAN_POINT('',(-0.0199671439070973,-0.599667668933546,0.325));
#38322=CARTESIAN_POINT('',(-1.11022302462516E-16,-0.565,0.06));
#38323=CARTESIAN_POINT('',(-1.11022302462516E-16,-0.565,0.06));
#38324=CARTESIAN_POINT('',(-1.11022302462516E-16,-0.565,0.59));
#38325=CARTESIAN_POINT('',(-1.11022302462516E-16,-0.565,0.06));
#38326=CARTESIAN_POINT('',(-1.11022302462516E-16,-0.565,0.59));
#38327=CARTESIAN_POINT('Origin',(-8.32667268468867E-17,-0.6025,0.59));
#38328=CARTESIAN_POINT('',(0.0199671439070971,-0.599667668933546,0.59));
#38329=CARTESIAN_POINT('Origin',(0.,0.,0.59));
#38330=CARTESIAN_POINT('',(0.0431968989868596,-0.64,0.59));
#38331=CARTESIAN_POINT('Origin',(0.0431968989868596,-0.64,0.06));
#38332=CARTESIAN_POINT('',(0.0199671439070971,-0.599667668933546,0.06));
#38333=CARTESIAN_POINT('',(0.019967143907097,-0.599667668933546,0.325));
#38334=CARTESIAN_POINT('',(0.0431968989868596,-0.64,0.06));
#38335=CARTESIAN_POINT('Origin',(-8.32667268468867E-17,-0.6025,0.06));
#38336=CARTESIAN_POINT('Origin',(0.,0.,0.06));
#38337=CARTESIAN_POINT('Origin',(-0.146232760482925,-0.545748091853324,
0.06));
#38338=CARTESIAN_POINT('',(-0.174492193429331,-0.574066611494015,0.06));
#38339=CARTESIAN_POINT('',(-0.174492193429331,-0.574066611494015,0.59));
#38340=CARTESIAN_POINT('',(-0.174492193429331,-0.574066611494015,0.325));
#38341=CARTESIAN_POINT('',(-0.146232760482925,-0.545748091853324,0.06));
#38342=CARTESIAN_POINT('',(-0.146232760482925,-0.545748091853324,0.06));
#38343=CARTESIAN_POINT('',(-0.146232760482925,-0.545748091853324,0.59));
#38344=CARTESIAN_POINT('',(-0.146232760482925,-0.545748091853324,0.06));
#38345=CARTESIAN_POINT('',(-0.146232760482925,-0.545748091853324,0.59));
#38346=CARTESIAN_POINT('Origin',(-0.155938474674269,-0.581970310339164,
0.59));
#38347=CARTESIAN_POINT('',(-0.13591863347514,-0.584402365732934,0.59));
#38348=CARTESIAN_POINT('Origin',(0.,0.,0.59));
#38349=CARTESIAN_POINT('',(-0.123919188518606,-0.629372708972173,0.59));
#38350=CARTESIAN_POINT('Origin',(-0.123919188518606,-0.629372708972173,
0.06));
#38351=CARTESIAN_POINT('',(-0.13591863347514,-0.584402365732934,0.06));
#38352=CARTESIAN_POINT('',(-0.13591863347514,-0.584402365732934,0.325));
#38353=CARTESIAN_POINT('',(-0.123919188518606,-0.629372708972173,0.06));
#38354=CARTESIAN_POINT('Origin',(-0.155938474674269,-0.581970310339164,
0.06));
#38355=CARTESIAN_POINT('Origin',(0.,0.,0.06));
#38356=CARTESIAN_POINT('Origin',(-0.2825,-0.489304353138208,0.06));
#38357=CARTESIAN_POINT('',(-0.317125888331339,-0.509343863171099,0.06));
#38358=CARTESIAN_POINT('',(-0.317125888331339,-0.509343863171099,0.59));
#38359=CARTESIAN_POINT('',(-0.317125888331339,-0.509343863171099,0.325));
#38360=CARTESIAN_POINT('',(-0.2825,-0.489304353138208,0.06));
#38361=CARTESIAN_POINT('',(-0.2825,-0.489304353138208,0.06));
#38362=CARTESIAN_POINT('',(-0.2825,-0.489304353138208,0.59));
#38363=CARTESIAN_POINT('',(-0.2825,-0.489304353138208,0.06));
#38364=CARTESIAN_POINT('',(-0.2825,-0.489304353138208,0.59));
#38365=CARTESIAN_POINT('Origin',(-0.30125,-0.521780305780124,0.59));
#38366=CARTESIAN_POINT('',(-0.282541780602208,-0.529311007078196,0.59));
#38367=CARTESIAN_POINT('Origin',(0.,0.,0.59));
#38368=CARTESIAN_POINT('',(-0.28259038811267,-0.57585470791547,0.59));
#38369=CARTESIAN_POINT('Origin',(-0.28259038811267,-0.57585470791547,0.06));
#38370=CARTESIAN_POINT('',(-0.282541780602208,-0.529311007078196,0.06));
#38371=CARTESIAN_POINT('',(-0.282541780602208,-0.529311007078196,0.325));
#38372=CARTESIAN_POINT('',(-0.28259038811267,-0.57585470791547,0.06));
#38373=CARTESIAN_POINT('Origin',(-0.30125,-0.521780305780124,0.06));
#38374=CARTESIAN_POINT('Origin',(0.,0.,0.06));
#38375=CARTESIAN_POINT('Origin',(-0.3995153313704,-0.399515331370399,0.06));
#38376=CARTESIAN_POINT('',(-0.438147978018877,-0.409910172303604,0.06));
#38377=CARTESIAN_POINT('',(-0.438147978018877,-0.409910172303604,0.59));
#38378=CARTESIAN_POINT('',(-0.438147978018876,-0.409910172303604,0.325));
#38379=CARTESIAN_POINT('',(-0.3995153313704,-0.399515331370399,0.06));
#38380=CARTESIAN_POINT('',(-0.3995153313704,-0.399515331370399,0.06));
#38381=CARTESIAN_POINT('',(-0.3995153313704,-0.399515331370399,0.59));
#38382=CARTESIAN_POINT('',(-0.3995153313704,-0.399515331370399,0.06));
#38383=CARTESIAN_POINT('',(-0.3995153313704,-0.399515331370399,0.59));
#38384=CARTESIAN_POINT('Origin',(-0.426031835664895,-0.426031835664895,
0.59));
#38385=CARTESIAN_POINT('',(-0.409910172303604,-0.438147978018876,0.59));
#38386=CARTESIAN_POINT('Origin',(0.,0.,0.59));
#38387=CARTESIAN_POINT('',(-0.422003519759552,-0.483093160159229,0.59));
#38388=CARTESIAN_POINT('Origin',(-0.422003519759552,-0.483093160159229,
0.06));
#38389=CARTESIAN_POINT('',(-0.409910172303604,-0.438147978018876,0.06));
#38390=CARTESIAN_POINT('',(-0.409910172303604,-0.438147978018876,0.325));
#38391=CARTESIAN_POINT('',(-0.422003519759552,-0.483093160159229,0.06));
#38392=CARTESIAN_POINT('Origin',(-0.426031835664895,-0.426031835664895,
0.06));
#38393=CARTESIAN_POINT('Origin',(0.,0.,0.06));
#38394=CARTESIAN_POINT('Origin',(-0.489304353138208,-0.2825,0.06));
#38395=CARTESIAN_POINT('',(-0.529311007078196,-0.282541780602207,0.06));
#38396=CARTESIAN_POINT('',(-0.529311007078196,-0.282541780602207,0.59));
#38397=CARTESIAN_POINT('',(-0.529311007078196,-0.282541780602207,0.325));
#38398=CARTESIAN_POINT('',(-0.489304353138208,-0.2825,0.06));
#38399=CARTESIAN_POINT('',(-0.489304353138208,-0.2825,0.06));
#38400=CARTESIAN_POINT('',(-0.489304353138208,-0.2825,0.59));
#38401=CARTESIAN_POINT('',(-0.489304353138208,-0.2825,0.06));
#38402=CARTESIAN_POINT('',(-0.489304353138208,-0.2825,0.59));
#38403=CARTESIAN_POINT('Origin',(-0.521780305780124,-0.30125,0.59));
#38404=CARTESIAN_POINT('',(-0.509343863171099,-0.317125888331339,0.59));
#38405=CARTESIAN_POINT('Origin',(0.,0.,0.59));
#38406=CARTESIAN_POINT('',(-0.532657808928611,-0.357409611887331,0.59));
#38407=CARTESIAN_POINT('Origin',(-0.532657808928611,-0.357409611887331,
0.06));
#38408=CARTESIAN_POINT('',(-0.509343863171099,-0.317125888331339,0.06));
#38409=CARTESIAN_POINT('',(-0.509343863171099,-0.317125888331339,0.325));
#38410=CARTESIAN_POINT('',(-0.532657808928611,-0.357409611887331,0.06));
#38411=CARTESIAN_POINT('Origin',(-0.521780305780124,-0.30125,0.06));
#38412=CARTESIAN_POINT('Origin',(0.,0.,0.06));
#38413=CARTESIAN_POINT('Origin',(-0.545748091853324,-0.146232760482924,
0.06));
#38414=CARTESIAN_POINT('',(-0.584402365732935,-0.135918633475139,0.06));
#38415=CARTESIAN_POINT('',(-0.584402365732935,-0.135918633475139,0.59));
#38416=CARTESIAN_POINT('',(-0.584402365732935,-0.135918633475139,0.325));
#38417=CARTESIAN_POINT('',(-0.545748091853324,-0.146232760482924,0.06));
#38418=CARTESIAN_POINT('',(-0.545748091853324,-0.146232760482924,0.06));
#38419=CARTESIAN_POINT('',(-0.545748091853324,-0.146232760482924,0.59));
#38420=CARTESIAN_POINT('',(-0.545748091853324,-0.146232760482924,0.06));
#38421=CARTESIAN_POINT('',(-0.545748091853324,-0.146232760482924,0.59));
#38422=CARTESIAN_POINT('Origin',(-0.581970310339164,-0.155938474674269,
0.59));
#38423=CARTESIAN_POINT('',(-0.574066611494016,-0.17449219342933,0.59));
#38424=CARTESIAN_POINT('Origin',(0.,0.,0.59));
#38425=CARTESIAN_POINT('',(-0.607012348677835,-0.207369189212621,0.59));
#38426=CARTESIAN_POINT('Origin',(-0.607012348677835,-0.207369189212621,
0.06));
#38427=CARTESIAN_POINT('',(-0.574066611494016,-0.17449219342933,0.06));
#38428=CARTESIAN_POINT('',(-0.574066611494016,-0.17449219342933,0.325));
#38429=CARTESIAN_POINT('',(-0.607012348677835,-0.207369189212621,0.06));
#38430=CARTESIAN_POINT('Origin',(-0.581970310339164,-0.155938474674269,
0.06));
#38431=CARTESIAN_POINT('Origin',(0.,0.,0.06));
#38432=CARTESIAN_POINT('Origin',(-0.565,8.32667268468867E-17,0.06));
#38433=CARTESIAN_POINT('',(-0.599667668933546,0.0199671439070973,0.06));
#38434=CARTESIAN_POINT('',(-0.599667668933546,0.0199671439070973,0.59));
#38435=CARTESIAN_POINT('',(-0.599667668933546,0.0199671439070973,0.325));
#38436=CARTESIAN_POINT('',(-0.565,8.32667268468867E-17,0.06));
#38437=CARTESIAN_POINT('',(-0.565,8.32667268468867E-17,0.06));
#38438=CARTESIAN_POINT('',(-0.565,8.32667268468867E-17,0.59));
#38439=CARTESIAN_POINT('',(-0.565,8.32667268468867E-17,0.06));
#38440=CARTESIAN_POINT('',(-0.565,8.32667268468867E-17,0.59));
#38441=CARTESIAN_POINT('Origin',(-0.6025,5.55111512312578E-17,0.59));
#38442=CARTESIAN_POINT('',(-0.6,-7.34788079488412E-17,0.59));
#38443=CARTESIAN_POINT('Origin',(0.,0.,0.59));
#38444=CARTESIAN_POINT('',(-0.599667668933546,-0.0199671439070971,0.59));
#38445=CARTESIAN_POINT('',(-0.64,-0.0431968989868596,0.59));
#38446=CARTESIAN_POINT('Origin',(0.,0.,0.59));
#38447=CARTESIAN_POINT('Origin',(-0.64,-0.0431968989868596,0.06));
#38448=CARTESIAN_POINT('',(-0.599667668933546,-0.0199671439070971,0.06));
#38449=CARTESIAN_POINT('',(-0.599667668933546,-0.019967143907097,0.325));
#38450=CARTESIAN_POINT('',(-0.64,-0.0431968989868596,0.06));
#38451=CARTESIAN_POINT('Origin',(-0.6025,5.55111512312578E-17,0.06));
#38452=CARTESIAN_POINT('',(-0.6,-7.34788079488412E-17,0.06));
#38453=CARTESIAN_POINT('Origin',(0.,0.,0.06));
#38454=CARTESIAN_POINT('Origin',(0.,0.,0.06));
#38455=CARTESIAN_POINT('Origin',(-0.545748091853324,0.146232760482924,0.06));
#38456=CARTESIAN_POINT('',(-0.574066611494016,0.174492193429331,0.06));
#38457=CARTESIAN_POINT('',(-0.574066611494016,0.174492193429331,0.59));
#38458=CARTESIAN_POINT('',(-0.574066611494016,0.174492193429331,0.325));
#38459=CARTESIAN_POINT('',(-0.545748091853324,0.146232760482924,0.06));
#38460=CARTESIAN_POINT('',(-0.545748091853324,0.146232760482924,0.06));
#38461=CARTESIAN_POINT('',(-0.545748091853324,0.146232760482924,0.59));
#38462=CARTESIAN_POINT('',(-0.545748091853324,0.146232760482924,0.06));
#38463=CARTESIAN_POINT('',(-0.545748091853324,0.146232760482924,0.59));
#38464=CARTESIAN_POINT('Origin',(-0.581970310339164,0.155938474674269,0.59));
#38465=CARTESIAN_POINT('',(-0.584402365732935,0.13591863347514,0.59));
#38466=CARTESIAN_POINT('Origin',(0.,0.,0.59));
#38467=CARTESIAN_POINT('',(-0.629372708972173,0.123919188518606,0.59));
#38468=CARTESIAN_POINT('Origin',(-0.629372708972173,0.123919188518606,0.06));
#38469=CARTESIAN_POINT('',(-0.584402365732935,0.13591863347514,0.06));
#38470=CARTESIAN_POINT('',(-0.584402365732934,0.13591863347514,0.325));
#38471=CARTESIAN_POINT('',(-0.629372708972173,0.123919188518606,0.06));
#38472=CARTESIAN_POINT('Origin',(-0.581970310339164,0.155938474674269,0.06));
#38473=CARTESIAN_POINT('Origin',(0.,0.,0.06));
#38474=CARTESIAN_POINT('Origin',(-0.489304353138208,0.2825,0.06));
#38475=CARTESIAN_POINT('',(-0.509343863171099,0.317125888331339,0.06));
#38476=CARTESIAN_POINT('',(-0.509343863171099,0.317125888331339,0.59));
#38477=CARTESIAN_POINT('',(-0.509343863171099,0.317125888331339,0.325));
#38478=CARTESIAN_POINT('',(-0.489304353138208,0.2825,0.06));
#38479=CARTESIAN_POINT('',(-0.489304353138208,0.2825,0.06));
#38480=CARTESIAN_POINT('',(-0.489304353138208,0.2825,0.59));
#38481=CARTESIAN_POINT('',(-0.489304353138208,0.2825,0.06));
#38482=CARTESIAN_POINT('',(-0.489304353138208,0.2825,0.59));
#38483=CARTESIAN_POINT('Origin',(-0.521780305780124,0.30125,0.59));
#38484=CARTESIAN_POINT('',(-0.529311007078196,0.282541780602208,0.59));
#38485=CARTESIAN_POINT('Origin',(0.,0.,0.59));
#38486=CARTESIAN_POINT('',(-0.57585470791547,0.28259038811267,0.59));
#38487=CARTESIAN_POINT('Origin',(-0.57585470791547,0.28259038811267,0.06));
#38488=CARTESIAN_POINT('',(-0.529311007078196,0.282541780602208,0.06));
#38489=CARTESIAN_POINT('',(-0.529311007078196,0.282541780602208,0.325));
#38490=CARTESIAN_POINT('',(-0.57585470791547,0.28259038811267,0.06));
#38491=CARTESIAN_POINT('Origin',(-0.521780305780124,0.30125,0.06));
#38492=CARTESIAN_POINT('Origin',(0.,0.,0.06));
#38493=CARTESIAN_POINT('Origin',(-0.399515331370399,0.399515331370399,0.06));
#38494=CARTESIAN_POINT('',(-0.409910172303604,0.438147978018876,0.06));
#38495=CARTESIAN_POINT('',(-0.409910172303604,0.438147978018876,0.59));
#38496=CARTESIAN_POINT('',(-0.409910172303604,0.438147978018876,0.325));
#38497=CARTESIAN_POINT('',(-0.399515331370399,0.399515331370399,0.06));
#38498=CARTESIAN_POINT('',(-0.399515331370399,0.399515331370399,0.06));
#38499=CARTESIAN_POINT('',(-0.399515331370399,0.399515331370399,0.59));
#38500=CARTESIAN_POINT('',(-0.399515331370399,0.399515331370399,0.06));
#38501=CARTESIAN_POINT('',(-0.399515331370399,0.399515331370399,0.59));
#38502=CARTESIAN_POINT('Origin',(-0.426031835664895,0.426031835664895,0.59));
#38503=CARTESIAN_POINT('',(-0.438147978018876,0.409910172303604,0.59));
#38504=CARTESIAN_POINT('Origin',(0.,0.,0.59));
#38505=CARTESIAN_POINT('',(-0.483093160159229,0.422003519759552,0.59));
#38506=CARTESIAN_POINT('Origin',(-0.483093160159229,0.422003519759552,0.06));
#38507=CARTESIAN_POINT('',(-0.438147978018876,0.409910172303604,0.06));
#38508=CARTESIAN_POINT('',(-0.438147978018876,0.409910172303604,0.325));
#38509=CARTESIAN_POINT('',(-0.483093160159229,0.422003519759552,0.06));
#38510=CARTESIAN_POINT('Origin',(-0.426031835664895,0.426031835664895,0.06));
#38511=CARTESIAN_POINT('Origin',(0.,0.,0.06));
#38512=CARTESIAN_POINT('Origin',(-0.2825,0.489304353138208,0.06));
#38513=CARTESIAN_POINT('',(-0.282541780602207,0.529311007078196,0.06));
#38514=CARTESIAN_POINT('',(-0.282541780602207,0.529311007078196,0.59));
#38515=CARTESIAN_POINT('',(-0.282541780602207,0.529311007078196,0.325));
#38516=CARTESIAN_POINT('',(-0.2825,0.489304353138208,0.06));
#38517=CARTESIAN_POINT('',(-0.2825,0.489304353138208,0.06));
#38518=CARTESIAN_POINT('',(-0.2825,0.489304353138208,0.59));
#38519=CARTESIAN_POINT('',(-0.2825,0.489304353138208,0.06));
#38520=CARTESIAN_POINT('',(-0.2825,0.489304353138208,0.59));
#38521=CARTESIAN_POINT('Origin',(-0.30125,0.521780305780125,0.59));
#38522=CARTESIAN_POINT('',(-0.317125888331339,0.509343863171099,0.59));
#38523=CARTESIAN_POINT('Origin',(0.,0.,0.59));
#38524=CARTESIAN_POINT('',(-0.357409611887331,0.532657808928611,0.59));
#38525=CARTESIAN_POINT('Origin',(-0.357409611887331,0.532657808928611,0.06));
#38526=CARTESIAN_POINT('',(-0.317125888331339,0.509343863171099,0.06));
#38527=CARTESIAN_POINT('',(-0.317125888331339,0.509343863171099,0.325));
#38528=CARTESIAN_POINT('',(-0.357409611887331,0.532657808928611,0.06));
#38529=CARTESIAN_POINT('Origin',(-0.30125,0.521780305780125,0.06));
#38530=CARTESIAN_POINT('Origin',(0.,0.,0.06));
#38531=CARTESIAN_POINT('Origin',(-0.146232760482924,0.545748091853324,0.06));
#38532=CARTESIAN_POINT('',(-0.135918633475139,0.584402365732935,0.06));
#38533=CARTESIAN_POINT('',(-0.135918633475139,0.584402365732935,0.59));
#38534=CARTESIAN_POINT('',(-0.135918633475139,0.584402365732935,0.325));
#38535=CARTESIAN_POINT('',(-0.146232760482924,0.545748091853324,0.06));
#38536=CARTESIAN_POINT('',(-0.146232760482924,0.545748091853324,0.06));
#38537=CARTESIAN_POINT('',(-0.146232760482924,0.545748091853324,0.59));
#38538=CARTESIAN_POINT('',(-0.146232760482924,0.545748091853324,0.06));
#38539=CARTESIAN_POINT('',(-0.146232760482924,0.545748091853324,0.59));
#38540=CARTESIAN_POINT('Origin',(-0.155938474674269,0.581970310339164,0.59));
#38541=CARTESIAN_POINT('',(-0.17449219342933,0.574066611494016,0.59));
#38542=CARTESIAN_POINT('Origin',(0.,0.,0.59));
#38543=CARTESIAN_POINT('',(-0.207369189212621,0.607012348677835,0.59));
#38544=CARTESIAN_POINT('Origin',(-0.207369189212621,0.607012348677835,0.06));
#38545=CARTESIAN_POINT('',(-0.17449219342933,0.574066611494016,0.06));
#38546=CARTESIAN_POINT('',(-0.17449219342933,0.574066611494016,0.325));
#38547=CARTESIAN_POINT('',(-0.207369189212621,0.607012348677835,0.06));
#38548=CARTESIAN_POINT('Origin',(-0.155938474674269,0.581970310339164,0.06));
#38549=CARTESIAN_POINT('Origin',(0.,0.,0.06));
#38550=CARTESIAN_POINT('Origin',(5.55111512312578E-17,0.565,0.06));
#38551=CARTESIAN_POINT('',(0.0199671439070973,0.599667668933546,0.06));
#38552=CARTESIAN_POINT('',(0.0199671439070973,0.599667668933546,0.59));
#38553=CARTESIAN_POINT('',(0.0199671439070972,0.599667668933546,0.325));
#38554=CARTESIAN_POINT('',(5.55111512312578E-17,0.565,0.06));
#38555=CARTESIAN_POINT('',(5.55111512312578E-17,0.565,0.06));
#38556=CARTESIAN_POINT('',(5.55111512312578E-17,0.565,0.59));
#38557=CARTESIAN_POINT('',(5.55111512312578E-17,0.565,0.06));
#38558=CARTESIAN_POINT('',(5.55111512312578E-17,0.565,0.59));
#38559=CARTESIAN_POINT('Origin',(2.77555756156289E-17,0.6025,0.59));
#38560=CARTESIAN_POINT('',(-0.0199671439070972,0.599667668933546,0.59));
#38561=CARTESIAN_POINT('Origin',(0.,0.,0.59));
#38562=CARTESIAN_POINT('',(-0.0431968989868596,0.64,0.59));
#38563=CARTESIAN_POINT('Origin',(-0.0431968989868596,0.64,0.06));
#38564=CARTESIAN_POINT('',(-0.0199671439070972,0.599667668933546,0.06));
#38565=CARTESIAN_POINT('',(-0.0199671439070972,0.599667668933546,0.325));
#38566=CARTESIAN_POINT('',(-0.0431968989868596,0.64,0.06));
#38567=CARTESIAN_POINT('Origin',(2.77555756156289E-17,0.6025,0.06));
#38568=CARTESIAN_POINT('Origin',(0.,0.,0.06));
#38569=CARTESIAN_POINT('Origin',(0.146232760482924,0.545748091853324,0.06));
#38570=CARTESIAN_POINT('',(0.174492193429331,0.574066611494016,0.06));
#38571=CARTESIAN_POINT('',(0.174492193429331,0.574066611494016,0.59));
#38572=CARTESIAN_POINT('',(0.174492193429331,0.574066611494016,0.325));
#38573=CARTESIAN_POINT('',(0.146232760482924,0.545748091853324,0.06));
#38574=CARTESIAN_POINT('',(0.146232760482924,0.545748091853324,0.06));
#38575=CARTESIAN_POINT('',(0.146232760482924,0.545748091853324,0.59));
#38576=CARTESIAN_POINT('',(0.146232760482924,0.545748091853324,0.06));
#38577=CARTESIAN_POINT('',(0.146232760482924,0.545748091853324,0.59));
#38578=CARTESIAN_POINT('Origin',(0.155938474674269,0.581970310339164,0.59));
#38579=CARTESIAN_POINT('',(0.13591863347514,0.584402365732935,0.59));
#38580=CARTESIAN_POINT('Origin',(0.,0.,0.59));
#38581=CARTESIAN_POINT('',(0.123919188518606,0.629372708972173,0.59));
#38582=CARTESIAN_POINT('Origin',(0.123919188518606,0.629372708972173,0.06));
#38583=CARTESIAN_POINT('',(0.13591863347514,0.584402365732935,0.06));
#38584=CARTESIAN_POINT('',(0.13591863347514,0.584402365732934,0.325));
#38585=CARTESIAN_POINT('',(0.123919188518606,0.629372708972173,0.06));
#38586=CARTESIAN_POINT('Origin',(0.155938474674269,0.581970310339164,0.06));
#38587=CARTESIAN_POINT('Origin',(0.,0.,0.06));
#38588=CARTESIAN_POINT('Origin',(0.2825,0.489304353138208,0.06));
#38589=CARTESIAN_POINT('',(0.317125888331339,0.509343863171099,0.06));
#38590=CARTESIAN_POINT('',(0.317125888331339,0.509343863171099,0.59));
#38591=CARTESIAN_POINT('',(0.317125888331339,0.509343863171099,0.325));
#38592=CARTESIAN_POINT('',(0.2825,0.489304353138208,0.06));
#38593=CARTESIAN_POINT('',(0.2825,0.489304353138208,0.06));
#38594=CARTESIAN_POINT('',(0.2825,0.489304353138208,0.59));
#38595=CARTESIAN_POINT('',(0.2825,0.489304353138208,0.06));
#38596=CARTESIAN_POINT('',(0.2825,0.489304353138208,0.59));
#38597=CARTESIAN_POINT('Origin',(0.30125,0.521780305780124,0.59));
#38598=CARTESIAN_POINT('',(0.282541780602207,0.529311007078196,0.59));
#38599=CARTESIAN_POINT('Origin',(0.,0.,0.59));
#38600=CARTESIAN_POINT('',(0.282590388112669,0.575854707915471,0.59));
#38601=CARTESIAN_POINT('Origin',(0.282590388112669,0.575854707915471,0.06));
#38602=CARTESIAN_POINT('',(0.282541780602207,0.529311007078196,0.06));
#38603=CARTESIAN_POINT('',(0.282541780602207,0.529311007078196,0.325));
#38604=CARTESIAN_POINT('',(0.282590388112669,0.575854707915471,0.06));
#38605=CARTESIAN_POINT('Origin',(0.30125,0.521780305780124,0.06));
#38606=CARTESIAN_POINT('Origin',(0.,0.,0.06));
#38607=CARTESIAN_POINT('Origin',(0.399515331370399,0.399515331370399,0.06));
#38608=CARTESIAN_POINT('',(0.438147978018876,0.409910172303604,0.06));
#38609=CARTESIAN_POINT('',(0.438147978018876,0.409910172303604,0.59));
#38610=CARTESIAN_POINT('',(0.438147978018876,0.409910172303604,0.325));
#38611=CARTESIAN_POINT('',(0.399515331370399,0.399515331370399,0.06));
#38612=CARTESIAN_POINT('',(0.399515331370399,0.399515331370399,0.06));
#38613=CARTESIAN_POINT('',(0.399515331370399,0.399515331370399,0.59));
#38614=CARTESIAN_POINT('',(0.399515331370399,0.399515331370399,0.06));
#38615=CARTESIAN_POINT('',(0.399515331370399,0.399515331370399,0.59));
#38616=CARTESIAN_POINT('Origin',(0.426031835664895,0.426031835664895,0.59));
#38617=CARTESIAN_POINT('',(0.409910172303604,0.438147978018876,0.59));
#38618=CARTESIAN_POINT('Origin',(0.,0.,0.59));
#38619=CARTESIAN_POINT('',(0.422003519759552,0.483093160159229,0.59));
#38620=CARTESIAN_POINT('Origin',(0.422003519759552,0.483093160159229,0.06));
#38621=CARTESIAN_POINT('',(0.409910172303604,0.438147978018876,0.06));
#38622=CARTESIAN_POINT('',(0.409910172303604,0.438147978018876,0.325));
#38623=CARTESIAN_POINT('',(0.422003519759552,0.483093160159229,0.06));
#38624=CARTESIAN_POINT('Origin',(0.426031835664895,0.426031835664895,0.06));
#38625=CARTESIAN_POINT('Origin',(0.,0.,0.06));
#38626=CARTESIAN_POINT('Origin',(0.489304353138208,0.2825,0.06));
#38627=CARTESIAN_POINT('',(0.529311007078196,0.282541780602207,0.06));
#38628=CARTESIAN_POINT('',(0.529311007078196,0.282541780602207,0.59));
#38629=CARTESIAN_POINT('',(0.529311007078196,0.282541780602207,0.325));
#38630=CARTESIAN_POINT('',(0.489304353138208,0.2825,0.06));
#38631=CARTESIAN_POINT('',(0.489304353138208,0.2825,0.06));
#38632=CARTESIAN_POINT('',(0.489304353138208,0.2825,0.59));
#38633=CARTESIAN_POINT('',(0.489304353138208,0.2825,0.06));
#38634=CARTESIAN_POINT('',(0.489304353138208,0.2825,0.59));
#38635=CARTESIAN_POINT('Origin',(0.521780305780124,0.30125,0.59));
#38636=CARTESIAN_POINT('',(0.509343863171099,0.317125888331339,0.59));
#38637=CARTESIAN_POINT('Origin',(0.,0.,0.59));
#38638=CARTESIAN_POINT('',(0.532657808928611,0.357409611887331,0.59));
#38639=CARTESIAN_POINT('Origin',(0.532657808928611,0.357409611887331,0.06));
#38640=CARTESIAN_POINT('',(0.509343863171099,0.317125888331339,0.06));
#38641=CARTESIAN_POINT('',(0.509343863171099,0.317125888331339,0.325));
#38642=CARTESIAN_POINT('',(0.532657808928611,0.357409611887331,0.06));
#38643=CARTESIAN_POINT('Origin',(0.521780305780124,0.30125,0.06));
#38644=CARTESIAN_POINT('Origin',(0.,0.,0.06));
#38645=CARTESIAN_POINT('Origin',(0.545748091853324,0.146232760482924,0.06));
#38646=CARTESIAN_POINT('',(0.584402365732935,0.135918633475139,0.06));
#38647=CARTESIAN_POINT('',(0.584402365732935,0.135918633475139,0.59));
#38648=CARTESIAN_POINT('',(0.584402365732935,0.135918633475139,0.325));
#38649=CARTESIAN_POINT('',(0.545748091853324,0.146232760482924,0.06));
#38650=CARTESIAN_POINT('',(0.545748091853324,0.146232760482924,0.06));
#38651=CARTESIAN_POINT('',(0.545748091853324,0.146232760482924,0.59));
#38652=CARTESIAN_POINT('',(0.545748091853324,0.146232760482924,0.06));
#38653=CARTESIAN_POINT('',(0.545748091853324,0.146232760482924,0.59));
#38654=CARTESIAN_POINT('Origin',(0.581970310339164,0.155938474674269,0.59));
#38655=CARTESIAN_POINT('',(0.574066611494016,0.17449219342933,0.59));
#38656=CARTESIAN_POINT('Origin',(0.,0.,0.59));
#38657=CARTESIAN_POINT('',(0.607012348677835,0.207369189212621,0.59));
#38658=CARTESIAN_POINT('Origin',(0.607012348677835,0.207369189212621,0.06));
#38659=CARTESIAN_POINT('',(0.574066611494016,0.17449219342933,0.06));
#38660=CARTESIAN_POINT('',(0.574066611494016,0.174492193429331,0.325));
#38661=CARTESIAN_POINT('',(0.607012348677835,0.207369189212621,0.06));
#38662=CARTESIAN_POINT('Origin',(0.581970310339164,0.155938474674269,0.06));
#38663=CARTESIAN_POINT('Origin',(0.,0.,0.06));
#38664=CARTESIAN_POINT('Origin',(0.565,0.,0.06));
#38665=CARTESIAN_POINT('',(0.599667668933546,-0.0199671439070972,0.06));
#38666=CARTESIAN_POINT('',(0.599667668933546,-0.0199671439070972,0.59));
#38667=CARTESIAN_POINT('',(0.599667668933546,-0.0199671439070972,0.325));
#38668=CARTESIAN_POINT('',(0.565,0.,0.06));
#38669=CARTESIAN_POINT('',(0.565,0.,0.06));
#38670=CARTESIAN_POINT('',(0.565,0.,0.59));
#38671=CARTESIAN_POINT('',(0.565,0.,0.06));
#38672=CARTESIAN_POINT('',(0.565,0.,0.59));
#38673=CARTESIAN_POINT('Origin',(0.6025,0.,0.59));
#38674=CARTESIAN_POINT('',(0.599667668933546,0.0199671439070972,0.59));
#38675=CARTESIAN_POINT('Origin',(0.,0.,0.59));
#38676=CARTESIAN_POINT('',(0.64,0.0431968989868597,0.59));
#38677=CARTESIAN_POINT('Origin',(0.64,0.0431968989868597,0.06));
#38678=CARTESIAN_POINT('',(0.599667668933546,0.0199671439070972,0.06));
#38679=CARTESIAN_POINT('',(0.599667668933546,0.0199671439070972,0.325));
#38680=CARTESIAN_POINT('',(0.64,0.0431968989868597,0.06));
#38681=CARTESIAN_POINT('Origin',(0.6025,0.,0.06));
#38682=CARTESIAN_POINT('Origin',(0.,0.,0.06));
#38683=CARTESIAN_POINT('Origin',(0.16,0.,-1.16));
#38684=CARTESIAN_POINT('',(-0.16,-1.95943487863577E-17,-1.16));
#38685=CARTESIAN_POINT('Origin',(0.,0.,-1.16));
#38686=CARTESIAN_POINT('Origin',(0.,0.,-1.14));
#38687=CARTESIAN_POINT('',(-0.18,-2.20436423846524E-17,-1.14));
#38688=CARTESIAN_POINT('Origin',(0.55,0.,0.));
#38689=CARTESIAN_POINT('',(-0.55,-6.73555739531044E-17,3.81639164714898E-17));
#38690=CARTESIAN_POINT('Origin',(0.,0.,0.));
#38691=CARTESIAN_POINT('Origin',(0.,0.,0.025));
#38692=CARTESIAN_POINT('',(-0.6,-7.34788079488412E-17,0.0500000000000001));
#38693=CARTESIAN_POINT('Origin',(0.,0.,0.05));
#38694=CARTESIAN_POINT('',(-0.575,-7.04171909509728E-17,0.025));
#38695=CARTESIAN_POINT('Origin',(0.,0.,0.325));
#38696=CARTESIAN_POINT('',(-0.6,-7.34788079488412E-17,0.6));
#38697=CARTESIAN_POINT('Origin',(0.,0.,0.6));
#38698=CARTESIAN_POINT('',(-0.6,-7.34788079488412E-17,0.325));
#38699=CARTESIAN_POINT('',(-0.6,-7.34788079488412E-17,0.325));
#38700=CARTESIAN_POINT('Origin',(0.,0.,0.65));
#38701=CARTESIAN_POINT('',(-0.5,-6.12323399573677E-17,0.7));
#38702=CARTESIAN_POINT('Origin',(0.,0.,0.7));
#38703=CARTESIAN_POINT('',(-0.55,-6.73555739531044E-17,0.65));
#38704=CARTESIAN_POINT('Origin',(0.,0.,0.7));
#53628=UNCERTAINTY_MEASURE_WITH_UNIT(LENGTH_MEASURE(0.001),#53651,
'DISTANCE_ACCURACY_VALUE',
'Maximum model space distance between geometric entities at asserted c
onnectivities');
#53632=UNCERTAINTY_MEASURE_WITH_UNIT(LENGTH_MEASURE(0.001),#53651,
'DISTANCE_ACCURACY_VALUE',
'Maximum model space distance between geometric entities at asserted c
onnectivities');
#53646=(
GEOMETRIC_REPRESENTATION_CONTEXT(3)
GLOBAL_UNCERTAINTY_ASSIGNED_CONTEXT((#53628))
GLOBAL_UNIT_ASSIGNED_CONTEXT((#53651,#53653,#53654))
REPRESENTATION_CONTEXT('','3D')
);
#53650=(
GEOMETRIC_REPRESENTATION_CONTEXT(3)
GLOBAL_UNCERTAINTY_ASSIGNED_CONTEXT((#53632))
GLOBAL_UNIT_ASSIGNED_CONTEXT((#53651,#53653,#53654))
REPRESENTATION_CONTEXT('','3D')
);
#53651=(
LENGTH_UNIT()
NAMED_UNIT(*)
SI_UNIT(.CENTI.,.METRE.)
);
#53653=(
NAMED_UNIT(*)
PLANE_ANGLE_UNIT()
SI_UNIT($,.RADIAN.)
);
#53654=(
NAMED_UNIT(*)
SI_UNIT($,.STERADIAN.)
SOLID_ANGLE_UNIT()
);
#53668=SHAPE_DEFINITION_REPRESENTATION(#53685,#53736);
#53685=PRODUCT_DEFINITION_SHAPE('',$,#53754);
#53736=SHAPE_REPRESENTATION('',(#24595),#53646);
#53740=PRODUCT_DEFINITION_CONTEXT('part definition',#53793,'design');
#53754=PRODUCT_DEFINITION('2026-10-18-22-44-46-618',
'11_Clip_Thumb_Knob_M4x12',#53771,#53740);
#53771=PRODUCT_DEFINITION_FORMATION('',$,#53808);
#53793=APPLICATION_CONTEXT(
'Core Data for Automotive Mechanical Design Process');
#53794=PRODUCT_CONTEXT('part definition',#53793,'mechanical');
#53808=PRODUCT('2026-10-18-22-44-46-618','11_Clip_Thumb_Knob_M4x12',$,(#53794));
#53938=COLOUR_RGB('Light Blue',0.38,0.62,0.78);
#53939=FILL_AREA_STYLE_COLOUR('',#53938);
#53940=FILL_AREA_STYLE('',(#53939));
#53941=SURFACE_STYLE_FILL_AREA(#53940);
#53942=SURFACE_SIDE_STYLE('',(#53941));
#53943=SURFACE_STYLE_USAGE(.BOTH.,#53942);
#53944=PRESENTATION_STYLE_ASSIGNMENT((#53943));
ENDSEC;
END-ISO-10303-21;
